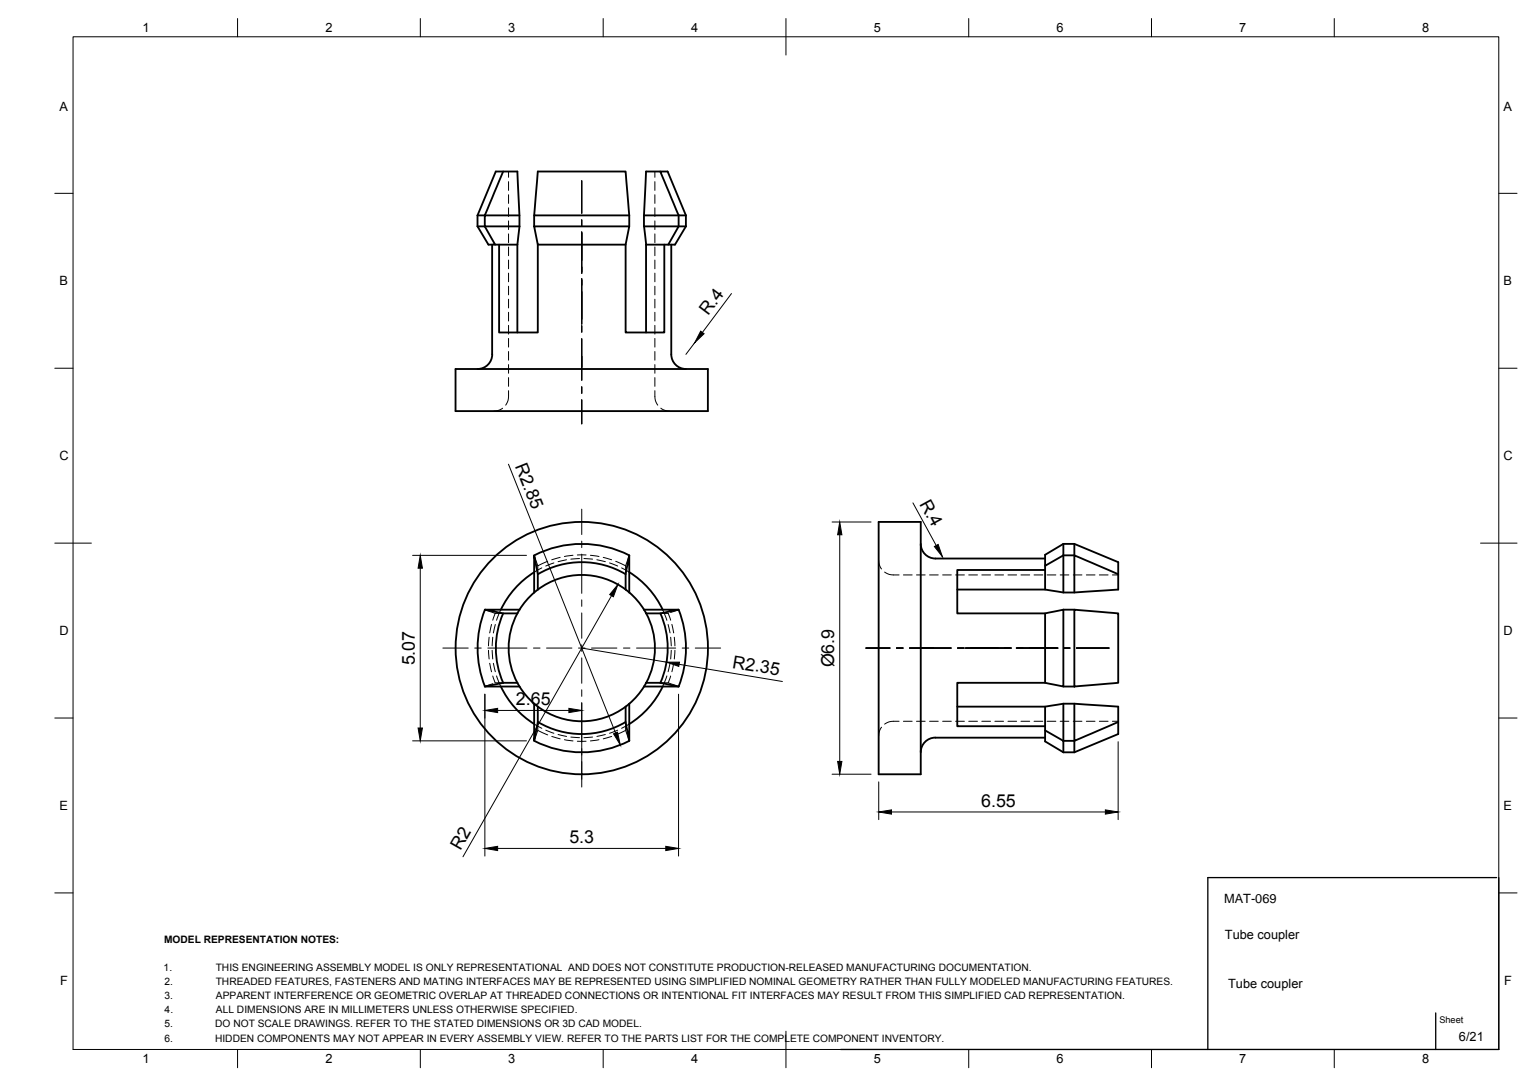
ISO-10303-21;
HEADER;
/* Generated by software containing ST-Developer
 * from STEP Tools, Inc. (www.steptools.com) 
 */

FILE_DESCRIPTION(
/* description */ ('CAx-IF Rec.Pracs.---Representation and Presentation of Product Manufa
cturing Information (PMI)---4.0---2014-10-13'),
/* implementation_level */ '2;1');

FILE_NAME(
/* name */ 'Tube coupler.step',
/* time_stamp */ '2026-10-24T15:08:39-07:00',
/* author */ (''),
/* organization */ (''),
/* preprocessor_version */ 'ST-DEVELOPER v20.2',
/* originating_system */ 'Autodesk Translation Framework v15.17.0.0',
/* authorisation */ '');

FILE_SCHEMA (('AP242_MANAGED_MODEL_BASED_3D_ENGINEERING_MIM_LF { 1 0 10303 442 2 1 4 }'));
ENDSEC;

DATA;
#10=MECHANICAL_DESIGN_GEOMETRIC_PRESENTATION_REPRESENTATION('',(#823),#50081);
#605=CONICAL_SURFACE('',#10189,0.0026,0.394791119699761);
#606=CONICAL_SURFACE('',#10204,0.0026,0.394791119699761);
#607=CONICAL_SURFACE('',#10207,0.0026,0.394791119699761);
#608=CONICAL_SURFACE('',#10215,0.0027,0.540419500270585);
#609=CONICAL_SURFACE('',#10219,0.0027,0.540419500270585);
#610=CONICAL_SURFACE('',#10227,0.0027,0.540419500270585);
#611=CONICAL_SURFACE('',#10235,0.0027,0.540419500270585);
#612=CONICAL_SURFACE('',#10257,0.0026,0.394791119699761);
#665=(
BOUNDED_CURVE()
B_SPLINE_CURVE(2,(#13666,#13667,#13668),.UNSPECIFIED.,.F.,.F.)
B_SPLINE_CURVE_WITH_KNOTS((3,3),(0.,0.130388293175992),.UNSPECIFIED.)
CURVE()
GEOMETRIC_REPRESENTATION_ITEM()
RATIONAL_B_SPLINE_CURVE((1.,1.00525170247464,1.))
REPRESENTATION_ITEM('')
);
#666=(
BOUNDED_CURVE()
B_SPLINE_CURVE(2,(#13674,#13675,#13676),.UNSPECIFIED.,.F.,.F.)
B_SPLINE_CURVE_WITH_KNOTS((3,3),(0.,0.130388293175992),.UNSPECIFIED.)
CURVE()
GEOMETRIC_REPRESENTATION_ITEM()
RATIONAL_B_SPLINE_CURVE((1.,1.00525170247464,1.))
REPRESENTATION_ITEM('')
);
#667=(
BOUNDED_CURVE()
B_SPLINE_CURVE(2,(#13686,#13687,#13688),.UNSPECIFIED.,.F.,.F.)
B_SPLINE_CURVE_WITH_KNOTS((3,3),(0.,0.1309950991442),.UNSPECIFIED.)
CURVE()
GEOMETRIC_REPRESENTATION_ITEM()
RATIONAL_B_SPLINE_CURVE((1.,1.00582981008257,1.))
REPRESENTATION_ITEM('')
);
#668=(
BOUNDED_CURVE()
B_SPLINE_CURVE(2,(#13697,#13698,#13699),.UNSPECIFIED.,.F.,.F.)
B_SPLINE_CURVE_WITH_KNOTS((3,3),(0.,0.1309950991442),.UNSPECIFIED.)
CURVE()
GEOMETRIC_REPRESENTATION_ITEM()
RATIONAL_B_SPLINE_CURVE((1.,1.00582981008257,1.))
REPRESENTATION_ITEM('')
);
#669=(
BOUNDED_CURVE()
B_SPLINE_CURVE(2,(#13708,#13709,#13710),.UNSPECIFIED.,.F.,.F.)
B_SPLINE_CURVE_WITH_KNOTS((3,3),(0.,0.1309950991442),.UNSPECIFIED.)
CURVE()
GEOMETRIC_REPRESENTATION_ITEM()
RATIONAL_B_SPLINE_CURVE((1.,1.00582981008257,1.))
REPRESENTATION_ITEM('')
);
#670=(
BOUNDED_CURVE()
B_SPLINE_CURVE(2,(#13715,#13716,#13717),.UNSPECIFIED.,.F.,.F.)
B_SPLINE_CURVE_WITH_KNOTS((3,3),(0.,0.130388293175992),.UNSPECIFIED.)
CURVE()
GEOMETRIC_REPRESENTATION_ITEM()
RATIONAL_B_SPLINE_CURVE((1.,1.00525170247464,1.))
REPRESENTATION_ITEM('')
);
#671=(
BOUNDED_CURVE()
B_SPLINE_CURVE(2,(#13727,#13728,#13729),.UNSPECIFIED.,.F.,.F.)
B_SPLINE_CURVE_WITH_KNOTS((3,3),(0.,0.130388293175992),.UNSPECIFIED.)
CURVE()
GEOMETRIC_REPRESENTATION_ITEM()
RATIONAL_B_SPLINE_CURVE((1.,1.00525170247464,1.))
REPRESENTATION_ITEM('')
);
#672=(
BOUNDED_CURVE()
B_SPLINE_CURVE(2,(#13732,#13733,#13734),.UNSPECIFIED.,.F.,.F.)
B_SPLINE_CURVE_WITH_KNOTS((3,3),(0.,0.1309950991442),.UNSPECIFIED.)
CURVE()
GEOMETRIC_REPRESENTATION_ITEM()
RATIONAL_B_SPLINE_CURVE((1.,1.00582981008257,1.))
REPRESENTATION_ITEM('')
);
#673=(
BOUNDED_CURVE()
B_SPLINE_CURVE(2,(#13762,#13763,#13764),.UNSPECIFIED.,.F.,.F.)
B_SPLINE_CURVE_WITH_KNOTS((3,3),(0.13740622471284,0.194564395432606),
 .UNSPECIFIED.)
CURVE()
GEOMETRIC_REPRESENTATION_ITEM()
RATIONAL_B_SPLINE_CURVE((1.0210752443686,1.02155284321629,1.018780946918))
REPRESENTATION_ITEM('')
);
#674=(
BOUNDED_CURVE()
B_SPLINE_CURVE(2,(#13772,#13773,#13774),.UNSPECIFIED.,.F.,.F.)
B_SPLINE_CURVE_WITH_KNOTS((3,3),(-0.194564395432341,-0.137406224712621),
 .UNSPECIFIED.)
CURVE()
GEOMETRIC_REPRESENTATION_ITEM()
RATIONAL_B_SPLINE_CURVE((1.01878094691633,1.02155284321435,1.02107524436669))
REPRESENTATION_ITEM('')
);
#675=(
BOUNDED_CURVE()
B_SPLINE_CURVE(2,(#13806,#13807,#13808),.UNSPECIFIED.,.F.,.F.)
B_SPLINE_CURVE_WITH_KNOTS((3,3),(0.137406224811474,0.19456439553049),
 .UNSPECIFIED.)
CURVE()
GEOMETRIC_REPRESENTATION_ITEM()
RATIONAL_B_SPLINE_CURVE((1.02107524478079,1.02155284363217,1.01878094727436))
REPRESENTATION_ITEM('')
);
#676=(
BOUNDED_CURVE()
B_SPLINE_CURVE(2,(#13815,#13816,#13817),.UNSPECIFIED.,.F.,.F.)
B_SPLINE_CURVE_WITH_KNOTS((3,3),(-0.194564395470828,-0.137406224751148),
 .UNSPECIFIED.)
CURVE()
GEOMETRIC_REPRESENTATION_ITEM()
RATIONAL_B_SPLINE_CURVE((1.01878094706027,1.02155284338227,1.02107524453305))
REPRESENTATION_ITEM('')
);
#687=ELLIPSE('',#10162,0.0240831891575954,0.00200000000001);
#688=ELLIPSE('',#10163,0.0101980390271974,0.00200000000001);
#689=ELLIPSE('',#10165,0.0101980390271974,0.00200000000001);
#690=ELLIPSE('',#10166,0.0240831891575954,0.00200000000001);
#691=ELLIPSE('',#10168,0.0240831891575954,0.00200000000001);
#692=ELLIPSE('',#10169,0.0101980390271974,0.00200000000001);
#693=ELLIPSE('',#10171,0.0101980390271974,0.00200000000001);
#694=ELLIPSE('',#10172,0.0240831891575954,0.00200000000001);
#695=ELLIPSE('',#10174,0.0240831891575954,0.00200000000001);
#696=ELLIPSE('',#10175,0.0101980390271974,0.00200000000001);
#697=ELLIPSE('',#10177,0.0101980390271974,0.00200000000001);
#698=ELLIPSE('',#10178,0.0240831891575954,0.00200000000001);
#699=ELLIPSE('',#10180,0.0240831891575954,0.00200000000001);
#700=ELLIPSE('',#10181,0.0101980390271974,0.00200000000001);
#701=ELLIPSE('',#10183,0.0101980390271974,0.00200000000001);
#702=ELLIPSE('',#10184,0.0240831891575954,0.00200000000001);
#710=FACE_BOUND('',#1658,.T.);
#711=FACE_BOUND('',#1663,.T.);
#771=TOROIDAL_SURFACE('',#10140,0.00285,0.0004);
#772=TOROIDAL_SURFACE('',#10156,0.0024,0.0004);
#783=SHAPE_REPRESENTATION_RELATIONSHIP('SRR','None',#50151,#803);
#803=ADVANCED_BREP_SHAPE_REPRESENTATION('',(#843),#50064);
#823=STYLED_ITEM('',(#50260),#843);
#843=MANIFOLD_SOLID_BREP('Body1',#9868);
#866=PLANE('',#10144);
#867=PLANE('',#10186);
#868=PLANE('',#10188);
#869=PLANE('',#10192);
#870=PLANE('',#10193);
#871=PLANE('',#10194);
#872=PLANE('',#10195);
#873=PLANE('',#10197);
#874=PLANE('',#10198);
#875=PLANE('',#10200);
#876=PLANE('',#10201);
#877=PLANE('',#10202);
#878=PLANE('',#10206);
#879=PLANE('',#10209);
#880=PLANE('',#10210);
#881=PLANE('',#10211);
#882=PLANE('',#10213);
#883=PLANE('',#10218);
#884=PLANE('',#10222);
#885=PLANE('',#10223);
#886=PLANE('',#10224);
#887=PLANE('',#10225);
#888=PLANE('',#10231);
#889=PLANE('',#10232);
#890=PLANE('',#10233);
#891=PLANE('',#10234);
#892=PLANE('',#10238);
#893=PLANE('',#10239);
#894=PLANE('',#10240);
#895=PLANE('',#10241);
#896=PLANE('',#10242);
#897=PLANE('',#10243);
#898=PLANE('',#10244);
#899=PLANE('',#10245);
#900=PLANE('',#10246);
#901=PLANE('',#10247);
#902=PLANE('',#10248);
#903=PLANE('',#10249);
#904=PLANE('',#10250);
#905=PLANE('',#10251);
#906=PLANE('',#10252);
#907=PLANE('',#10254);
#908=PLANE('',#10256);
#909=PLANE('',#10260);
#910=PLANE('',#10262);
#911=PLANE('',#10264);
#1115=FACE_OUTER_BOUND('',#1656,.T.);
#1116=FACE_OUTER_BOUND('',#1657,.T.);
#1117=FACE_OUTER_BOUND('',#1659,.T.);
#1118=FACE_OUTER_BOUND('',#1660,.T.);
#1119=FACE_OUTER_BOUND('',#1661,.T.);
#1120=FACE_OUTER_BOUND('',#1662,.T.);
#1121=FACE_OUTER_BOUND('',#1664,.T.);
#1122=FACE_OUTER_BOUND('',#1665,.T.);
#1123=FACE_OUTER_BOUND('',#1666,.T.);
#1124=FACE_OUTER_BOUND('',#1667,.T.);
#1125=FACE_OUTER_BOUND('',#1668,.T.);
#1126=FACE_OUTER_BOUND('',#1669,.T.);
#1127=FACE_OUTER_BOUND('',#1670,.T.);
#1128=FACE_OUTER_BOUND('',#1671,.T.);
#1129=FACE_OUTER_BOUND('',#1672,.T.);
#1130=FACE_OUTER_BOUND('',#1673,.T.);
#1131=FACE_OUTER_BOUND('',#1674,.T.);
#1132=FACE_OUTER_BOUND('',#1675,.T.);
#1133=FACE_OUTER_BOUND('',#1676,.T.);
#1134=FACE_OUTER_BOUND('',#1677,.T.);
#1135=FACE_OUTER_BOUND('',#1678,.T.);
#1136=FACE_OUTER_BOUND('',#1679,.T.);
#1137=FACE_OUTER_BOUND('',#1680,.T.);
#1138=FACE_OUTER_BOUND('',#1681,.T.);
#1139=FACE_OUTER_BOUND('',#1682,.T.);
#1140=FACE_OUTER_BOUND('',#1683,.T.);
#1141=FACE_OUTER_BOUND('',#1684,.T.);
#1142=FACE_OUTER_BOUND('',#1685,.T.);
#1143=FACE_OUTER_BOUND('',#1686,.T.);
#1144=FACE_OUTER_BOUND('',#1687,.T.);
#1145=FACE_OUTER_BOUND('',#1688,.T.);
#1146=FACE_OUTER_BOUND('',#1689,.T.);
#1147=FACE_OUTER_BOUND('',#1690,.T.);
#1148=FACE_OUTER_BOUND('',#1691,.T.);
#1149=FACE_OUTER_BOUND('',#1692,.T.);
#1150=FACE_OUTER_BOUND('',#1693,.T.);
#1151=FACE_OUTER_BOUND('',#1694,.T.);
#1152=FACE_OUTER_BOUND('',#1695,.T.);
#1153=FACE_OUTER_BOUND('',#1696,.T.);
#1154=FACE_OUTER_BOUND('',#1697,.T.);
#1155=FACE_OUTER_BOUND('',#1698,.T.);
#1156=FACE_OUTER_BOUND('',#1699,.T.);
#1157=FACE_OUTER_BOUND('',#1700,.T.);
#1158=FACE_OUTER_BOUND('',#1701,.T.);
#1159=FACE_OUTER_BOUND('',#1702,.T.);
#1160=FACE_OUTER_BOUND('',#1703,.T.);
#1161=FACE_OUTER_BOUND('',#1704,.T.);
#1162=FACE_OUTER_BOUND('',#1705,.T.);
#1163=FACE_OUTER_BOUND('',#1706,.T.);
#1164=FACE_OUTER_BOUND('',#1707,.T.);
#1165=FACE_OUTER_BOUND('',#1708,.T.);
#1166=FACE_OUTER_BOUND('',#1709,.T.);
#1167=FACE_OUTER_BOUND('',#1710,.T.);
#1168=FACE_OUTER_BOUND('',#1711,.T.);
#1169=FACE_OUTER_BOUND('',#1712,.T.);
#1170=FACE_OUTER_BOUND('',#1713,.T.);
#1171=FACE_OUTER_BOUND('',#1714,.T.);
#1172=FACE_OUTER_BOUND('',#1715,.T.);
#1173=FACE_OUTER_BOUND('',#1716,.T.);
#1174=FACE_OUTER_BOUND('',#1717,.T.);
#1175=FACE_OUTER_BOUND('',#1718,.T.);
#1176=FACE_OUTER_BOUND('',#1719,.T.);
#1177=FACE_OUTER_BOUND('',#1720,.T.);
#1656=EDGE_LOOP('',(#6268,#6269,#6270,#6271));
#1657=EDGE_LOOP('',(#6272));
#1658=EDGE_LOOP('',(#6273));
#1659=EDGE_LOOP('',(#6274,#6275,#6276,#6277,#6278,#6279,#6280,#6281,#6282,
#6283,#6284,#6285,#6286,#6287,#6288,#6289,#6290,#6291,#6292,#6293));
#1660=EDGE_LOOP('',(#6294,#6295,#6296,#6297));
#1661=EDGE_LOOP('',(#6298,#6299,#6300,#6301,#6302,#6303,#6304,#6305,#6306,
#6307,#6308,#6309,#6310,#6311,#6312,#6313,#6314,#6315,#6316,#6317,#6318,
#6319,#6320,#6321,#6322,#6323,#6324,#6325,#6326,#6327,#6328,#6329,#6330,
#6331,#6332,#6333,#6334,#6335,#6336,#6337,#6338,#6339,#6340,#6341));
#1662=EDGE_LOOP('',(#6342));
#1663=EDGE_LOOP('',(#6343));
#1664=EDGE_LOOP('',(#6344,#6345,#6346,#6347));
#1665=EDGE_LOOP('',(#6348,#6349,#6350,#6351));
#1666=EDGE_LOOP('',(#6352,#6353,#6354,#6355));
#1667=EDGE_LOOP('',(#6356,#6357,#6358,#6359));
#1668=EDGE_LOOP('',(#6360,#6361,#6362,#6363));
#1669=EDGE_LOOP('',(#6364,#6365,#6366,#6367));
#1670=EDGE_LOOP('',(#6368,#6369,#6370,#6371));
#1671=EDGE_LOOP('',(#6372,#6373,#6374,#6375,#6376));
#1672=EDGE_LOOP('',(#6377,#6378,#6379,#6380));
#1673=EDGE_LOOP('',(#6381,#6382,#6383,#6384));
#1674=EDGE_LOOP('',(#6385,#6386,#6387,#6388));
#1675=EDGE_LOOP('',(#6389,#6390,#6391,#6392));
#1676=EDGE_LOOP('',(#6393,#6394,#6395,#6396));
#1677=EDGE_LOOP('',(#6397,#6398,#6399,#6400));
#1678=EDGE_LOOP('',(#6401,#6402,#6403,#6404));
#1679=EDGE_LOOP('',(#6405,#6406,#6407,#6408));
#1680=EDGE_LOOP('',(#6409,#6410,#6411,#6412,#6413));
#1681=EDGE_LOOP('',(#6414,#6415,#6416,#6417));
#1682=EDGE_LOOP('',(#6418,#6419,#6420,#6421));
#1683=EDGE_LOOP('',(#6422,#6423,#6424,#6425,#6426));
#1684=EDGE_LOOP('',(#6427,#6428,#6429,#6430));
#1685=EDGE_LOOP('',(#6431,#6432,#6433,#6434));
#1686=EDGE_LOOP('',(#6435,#6436,#6437,#6438,#6439));
#1687=EDGE_LOOP('',(#6440,#6441,#6442,#6443));
#1688=EDGE_LOOP('',(#6444,#6445,#6446,#6447,#6448));
#1689=EDGE_LOOP('',(#6449,#6450,#6451,#6452));
#1690=EDGE_LOOP('',(#6453,#6454,#6455,#6456,#6457));
#1691=EDGE_LOOP('',(#6458,#6459,#6460,#6461,#6462));
#1692=EDGE_LOOP('',(#6463,#6464,#6465,#6466));
#1693=EDGE_LOOP('',(#6467,#6468,#6469,#6470,#6471));
#1694=EDGE_LOOP('',(#6472,#6473,#6474,#6475));
#1695=EDGE_LOOP('',(#6476,#6477,#6478,#6479));
#1696=EDGE_LOOP('',(#6480,#6481,#6482,#6483,#6484));
#1697=EDGE_LOOP('',(#6485,#6486,#6487,#6488,#6489));
#1698=EDGE_LOOP('',(#6490,#6491,#6492,#6493));
#1699=EDGE_LOOP('',(#6494,#6495,#6496,#6497));
#1700=EDGE_LOOP('',(#6498,#6499,#6500,#6501));
#1701=EDGE_LOOP('',(#6502,#6503,#6504,#6505));
#1702=EDGE_LOOP('',(#6506,#6507,#6508,#6509));
#1703=EDGE_LOOP('',(#6510,#6511,#6512,#6513));
#1704=EDGE_LOOP('',(#6514,#6515,#6516,#6517));
#1705=EDGE_LOOP('',(#6518,#6519,#6520,#6521));
#1706=EDGE_LOOP('',(#6522,#6523,#6524,#6525));
#1707=EDGE_LOOP('',(#6526,#6527,#6528,#6529));
#1708=EDGE_LOOP('',(#6530,#6531,#6532,#6533));
#1709=EDGE_LOOP('',(#6534,#6535,#6536,#6537));
#1710=EDGE_LOOP('',(#6538,#6539,#6540,#6541));
#1711=EDGE_LOOP('',(#6542,#6543,#6544,#6545));
#1712=EDGE_LOOP('',(#6546,#6547,#6548,#6549));
#1713=EDGE_LOOP('',(#6550,#6551,#6552,#6553));
#1714=EDGE_LOOP('',(#6554,#6555,#6556,#6557));
#1715=EDGE_LOOP('',(#6558,#6559,#6560,#6561));
#1716=EDGE_LOOP('',(#6562,#6563,#6564,#6565));
#1717=EDGE_LOOP('',(#6566,#6567,#6568,#6569));
#1718=EDGE_LOOP('',(#6570,#6571,#6572,#6573));
#1719=EDGE_LOOP('',(#6574,#6575,#6576,#6577));
#1720=EDGE_LOOP('',(#6578,#6579,#6580,#6581));
#2248=LINE('',#13538,#2826);
#2249=LINE('',#13542,#2827);
#2250=LINE('',#13546,#2828);
#2251=LINE('',#13550,#2829);
#2252=LINE('',#13554,#2830);
#2253=LINE('',#13558,#2831);
#2254=LINE('',#13562,#2832);
#2255=LINE('',#13566,#2833);
#2256=LINE('',#13568,#2834);
#2257=LINE('',#13577,#2835);
#2258=LINE('',#13583,#2836);
#2259=LINE('',#13587,#2837);
#2260=LINE('',#13591,#2838);
#2261=LINE('',#13595,#2839);
#2262=LINE('',#13603,#2840);
#2263=LINE('',#13607,#2841);
#2264=LINE('',#13611,#2842);
#2265=LINE('',#13615,#2843);
#2266=LINE('',#13623,#2844);
#2267=LINE('',#13627,#2845);
#2268=LINE('',#13631,#2846);
#2269=LINE('',#13635,#2847);
#2270=LINE('',#13643,#2848);
#2271=LINE('',#13647,#2849);
#2272=LINE('',#13651,#2850);
#2273=LINE('',#13655,#2851);
#2274=LINE('',#13664,#2852);
#2275=LINE('',#13669,#2853);
#2276=LINE('',#13679,#2854);
#2277=LINE('',#13681,#2855);
#2278=LINE('',#13684,#2856);
#2279=LINE('',#13689,#2857);
#2280=LINE('',#13692,#2858);
#2281=LINE('',#13700,#2859);
#2282=LINE('',#13701,#2860);
#2283=LINE('',#13705,#2861);
#2284=LINE('',#13711,#2862);
#2285=LINE('',#13718,#2863);
#2286=LINE('',#13719,#2864);
#2287=LINE('',#13723,#2865);
#2288=LINE('',#13735,#2866);
#2289=LINE('',#13739,#2867);
#2290=LINE('',#13742,#2868);
#2291=LINE('',#13743,#2869);
#2292=LINE('',#13746,#2870);
#2293=LINE('',#13749,#2871);
#2294=LINE('',#13750,#2872);
#2295=LINE('',#13754,#2873);
#2296=LINE('',#13765,#2874);
#2297=LINE('',#13766,#2875);
#2298=LINE('',#13767,#2876);
#2299=LINE('',#13777,#2877);
#2300=LINE('',#13779,#2878);
#2301=LINE('',#13780,#2879);
#2302=LINE('',#13782,#2880);
#2303=LINE('',#13787,#2881);
#2304=LINE('',#13788,#2882);
#2305=LINE('',#13789,#2883);
#2306=LINE('',#13797,#2884);
#2307=LINE('',#13799,#2885);
#2308=LINE('',#13800,#2886);
#2309=LINE('',#13802,#2887);
#2310=LINE('',#13809,#2888);
#2311=LINE('',#13810,#2889);
#2312=LINE('',#13811,#2890);
#2313=LINE('',#13820,#2891);
#2314=LINE('',#13822,#2892);
#2315=LINE('',#13823,#2893);
#2316=LINE('',#13825,#2894);
#2317=LINE('',#13827,#2895);
#2318=LINE('',#13829,#2896);
#2319=LINE('',#13831,#2897);
#2320=LINE('',#13833,#2898);
#2321=LINE('',#13835,#2899);
#2322=LINE('',#13837,#2900);
#2323=LINE('',#13839,#2901);
#2324=LINE('',#13841,#2902);
#2325=LINE('',#13847,#2903);
#2326=LINE('',#13849,#2904);
#2327=LINE('',#13851,#2905);
#2328=LINE('',#13856,#2906);
#2329=LINE('',#13859,#2907);
#2330=LINE('',#13862,#2908);
#2826=VECTOR('',#11124,1.);
#2827=VECTOR('',#11127,1.);
#2828=VECTOR('',#11130,1.);
#2829=VECTOR('',#11133,1.);
#2830=VECTOR('',#11136,1.);
#2831=VECTOR('',#11139,1.);
#2832=VECTOR('',#11142,1.);
#2833=VECTOR('',#11145,1.);
#2834=VECTOR('',#11148,0.00245);
#2835=VECTOR('',#11159,0.002);
#2836=VECTOR('',#11164,1.);
#2837=VECTOR('',#11167,1.);
#2838=VECTOR('',#11170,1.);
#2839=VECTOR('',#11173,1.);
#2840=VECTOR('',#11180,1.);
#2841=VECTOR('',#11183,1.);
#2842=VECTOR('',#11186,1.);
#2843=VECTOR('',#11189,1.);
#2844=VECTOR('',#11196,1.);
#2845=VECTOR('',#11199,1.);
#2846=VECTOR('',#11202,1.);
#2847=VECTOR('',#11205,1.);
#2848=VECTOR('',#11212,1.);
#2849=VECTOR('',#11215,1.);
#2850=VECTOR('',#11218,1.);
#2851=VECTOR('',#11221,1.);
#2852=VECTOR('',#11232,1.);
#2853=VECTOR('',#11233,1.);
#2854=VECTOR('',#11242,1.);
#2855=VECTOR('',#11245,1.);
#2856=VECTOR('',#11248,1.);
#2857=VECTOR('',#11249,1.);
#2858=VECTOR('',#11252,1.);
#2859=VECTOR('',#11257,1.);
#2860=VECTOR('',#11258,1.);
#2861=VECTOR('',#11263,1.);
#2862=VECTOR('',#11266,1.);
#2863=VECTOR('',#11269,1.);
#2864=VECTOR('',#11270,1.);
#2865=VECTOR('',#11275,1.);
#2866=VECTOR('',#11282,1.);
#2867=VECTOR('',#11289,1.);
#2868=VECTOR('',#11292,1.);
#2869=VECTOR('',#11293,1.);
#2870=VECTOR('',#11296,1.);
#2871=VECTOR('',#11299,1.);
#2872=VECTOR('',#11300,1.);
#2873=VECTOR('',#11305,1.);
#2874=VECTOR('',#11314,1.);
#2875=VECTOR('',#11315,1.);
#2876=VECTOR('',#11316,1.);
#2877=VECTOR('',#11325,1.);
#2878=VECTOR('',#11328,1.);
#2879=VECTOR('',#11329,1.);
#2880=VECTOR('',#11332,1.);
#2881=VECTOR('',#11337,1.);
#2882=VECTOR('',#11338,1.);
#2883=VECTOR('',#11339,1.);
#2884=VECTOR('',#11350,1.);
#2885=VECTOR('',#11353,1.);
#2886=VECTOR('',#11354,1.);
#2887=VECTOR('',#11357,1.);
#2888=VECTOR('',#11360,1.);
#2889=VECTOR('',#11361,1.);
#2890=VECTOR('',#11362,1.);
#2891=VECTOR('',#11371,1.);
#2892=VECTOR('',#11374,1.);
#2893=VECTOR('',#11375,1.);
#2894=VECTOR('',#11378,1.);
#2895=VECTOR('',#11381,1.);
#2896=VECTOR('',#11384,1.);
#2897=VECTOR('',#11387,1.);
#2898=VECTOR('',#11390,1.);
#2899=VECTOR('',#11393,1.);
#2900=VECTOR('',#11396,1.);
#2901=VECTOR('',#11399,1.);
#2902=VECTOR('',#11402,1.);
#2903=VECTOR('',#11413,0.00345);
#2904=VECTOR('',#11416,1.);
#2905=VECTOR('',#11419,1.);
#2906=VECTOR('',#11428,1.);
#2907=VECTOR('',#11433,1.);
#2908=VECTOR('',#11438,1.);
#3415=CIRCLE('',#10141,0.0028500000000131);
#3416=CIRCLE('',#10142,0.0004);
#3417=CIRCLE('',#10143,0.00245000000001309);
#3418=CIRCLE('',#10145,0.00345000000001);
#3419=CIRCLE('',#10147,0.00245000000001);
#3420=CIRCLE('',#10148,0.00245000000001);
#3421=CIRCLE('',#10149,0.00245000000001);
#3422=CIRCLE('',#10150,0.00245000000001);
#3423=CIRCLE('',#10151,0.00245000000001);
#3424=CIRCLE('',#10152,0.00245000000001);
#3425=CIRCLE('',#10153,0.00245000000001);
#3426=CIRCLE('',#10154,0.00245000000001);
#3427=CIRCLE('',#10155,0.00245000000001);
#3428=CIRCLE('',#10157,0.00200000000001);
#3429=CIRCLE('',#10158,0.0004);
#3430=CIRCLE('',#10159,0.00240000000001);
#3431=CIRCLE('',#10161,0.00200000000001);
#3432=CIRCLE('',#10164,0.00200000000001);
#3433=CIRCLE('',#10167,0.00200000000001);
#3434=CIRCLE('',#10170,0.00200000000001);
#3435=CIRCLE('',#10173,0.00200000000001);
#3436=CIRCLE('',#10176,0.00200000000001);
#3437=CIRCLE('',#10179,0.00200000000001);
#3438=CIRCLE('',#10182,0.00200000000001);
#3439=CIRCLE('',#10185,0.00200000000001);
#3440=CIRCLE('',#10187,0.00345000000001);
#3441=CIRCLE('',#10190,0.00235000000001);
#3442=CIRCLE('',#10191,0.00285000000001);
#3443=CIRCLE('',#10196,0.00235000000001);
#3444=CIRCLE('',#10199,0.00235000000001);
#3445=CIRCLE('',#10203,0.00235000000001);
#3446=CIRCLE('',#10205,0.00285000000001);
#3447=CIRCLE('',#10208,0.00285000000001);
#3448=CIRCLE('',#10212,0.481704687282423);
#3449=CIRCLE('',#10214,0.00255000000001);
#3450=CIRCLE('',#10216,0.00285000000001);
#3451=CIRCLE('',#10217,0.481704687282423);
#3452=CIRCLE('',#10220,0.00255000000001);
#3453=CIRCLE('',#10221,0.00285000000001);
#3454=CIRCLE('',#10226,0.481704687282423);
#3455=CIRCLE('',#10228,0.00255000000001);
#3456=CIRCLE('',#10229,0.481704687282423);
#3457=CIRCLE('',#10230,0.00285000000001);
#3458=CIRCLE('',#10236,0.00255000000001);
#3459=CIRCLE('',#10237,0.00285000000001);
#3460=CIRCLE('',#10258,0.00285000000001);
#3786=VERTEX_POINT('',#13525);
#3787=VERTEX_POINT('',#13527);
#3788=VERTEX_POINT('',#13531);
#3789=VERTEX_POINT('',#13534);
#3790=VERTEX_POINT('',#13535);
#3791=VERTEX_POINT('',#13537);
#3792=VERTEX_POINT('',#13539);
#3793=VERTEX_POINT('',#13541);
#3794=VERTEX_POINT('',#13543);
#3795=VERTEX_POINT('',#13545);
#3796=VERTEX_POINT('',#13547);
#3797=VERTEX_POINT('',#13549);
#3798=VERTEX_POINT('',#13551);
#3799=VERTEX_POINT('',#13553);
#3800=VERTEX_POINT('',#13555);
#3801=VERTEX_POINT('',#13557);
#3802=VERTEX_POINT('',#13559);
#3803=VERTEX_POINT('',#13561);
#3804=VERTEX_POINT('',#13563);
#3805=VERTEX_POINT('',#13565);
#3806=VERTEX_POINT('',#13570);
#3807=VERTEX_POINT('',#13572);
#3808=VERTEX_POINT('',#13576);
#3809=VERTEX_POINT('',#13578);
#3810=VERTEX_POINT('',#13580);
#3811=VERTEX_POINT('',#13582);
#3812=VERTEX_POINT('',#13584);
#3813=VERTEX_POINT('',#13586);
#3814=VERTEX_POINT('',#13588);
#3815=VERTEX_POINT('',#13590);
#3816=VERTEX_POINT('',#13592);
#3817=VERTEX_POINT('',#13594);
#3818=VERTEX_POINT('',#13596);
#3819=VERTEX_POINT('',#13598);
#3820=VERTEX_POINT('',#13600);
#3821=VERTEX_POINT('',#13602);
#3822=VERTEX_POINT('',#13604);
#3823=VERTEX_POINT('',#13606);
#3824=VERTEX_POINT('',#13608);
#3825=VERTEX_POINT('',#13610);
#3826=VERTEX_POINT('',#13612);
#3827=VERTEX_POINT('',#13614);
#3828=VERTEX_POINT('',#13616);
#3829=VERTEX_POINT('',#13618);
#3830=VERTEX_POINT('',#13620);
#3831=VERTEX_POINT('',#13622);
#3832=VERTEX_POINT('',#13624);
#3833=VERTEX_POINT('',#13626);
#3834=VERTEX_POINT('',#13628);
#3835=VERTEX_POINT('',#13630);
#3836=VERTEX_POINT('',#13632);
#3837=VERTEX_POINT('',#13634);
#3838=VERTEX_POINT('',#13636);
#3839=VERTEX_POINT('',#13638);
#3840=VERTEX_POINT('',#13640);
#3841=VERTEX_POINT('',#13642);
#3842=VERTEX_POINT('',#13644);
#3843=VERTEX_POINT('',#13646);
#3844=VERTEX_POINT('',#13648);
#3845=VERTEX_POINT('',#13650);
#3846=VERTEX_POINT('',#13652);
#3847=VERTEX_POINT('',#13654);
#3848=VERTEX_POINT('',#13656);
#3849=VERTEX_POINT('',#13660);
#3850=VERTEX_POINT('',#13663);
#3851=VERTEX_POINT('',#13665);
#3852=VERTEX_POINT('',#13671);
#3853=VERTEX_POINT('',#13673);
#3854=VERTEX_POINT('',#13683);
#3855=VERTEX_POINT('',#13685);
#3856=VERTEX_POINT('',#13691);
#3857=VERTEX_POINT('',#13695);
#3858=VERTEX_POINT('',#13696);
#3859=VERTEX_POINT('',#13703);
#3860=VERTEX_POINT('',#13707);
#3861=VERTEX_POINT('',#13713);
#3862=VERTEX_POINT('',#13714);
#3863=VERTEX_POINT('',#13721);
#3864=VERTEX_POINT('',#13725);
#3865=VERTEX_POINT('',#13731);
#3866=VERTEX_POINT('',#13741);
#3867=VERTEX_POINT('',#13745);
#3868=VERTEX_POINT('',#13747);
#3869=VERTEX_POINT('',#13752);
#3870=VERTEX_POINT('',#13756);
#3871=VERTEX_POINT('',#13760);
#3872=VERTEX_POINT('',#13761);
#3873=VERTEX_POINT('',#13769);
#3874=VERTEX_POINT('',#13771);
#3875=VERTEX_POINT('',#13784);
#3876=VERTEX_POINT('',#13785);
#3877=VERTEX_POINT('',#13791);
#3878=VERTEX_POINT('',#13793);
#3879=VERTEX_POINT('',#13804);
#3880=VERTEX_POINT('',#13805);
#3881=VERTEX_POINT('',#13813);
#4787=EDGE_CURVE('',#3786,#3786,#3415,.T.);
#4788=EDGE_CURVE('',#3786,#3787,#3416,.T.);
#4789=EDGE_CURVE('',#3787,#3787,#3417,.T.);
#4790=EDGE_CURVE('',#3788,#3788,#3418,.T.);
#4791=EDGE_CURVE('',#3789,#3790,#3419,.T.);
#4792=EDGE_CURVE('',#3791,#3789,#2248,.T.);
#4793=EDGE_CURVE('',#3792,#3791,#3420,.T.);
#4794=EDGE_CURVE('',#3792,#3793,#2249,.T.);
#4795=EDGE_CURVE('',#3794,#3793,#3421,.T.);
#4796=EDGE_CURVE('',#3795,#3794,#2250,.T.);
#4797=EDGE_CURVE('',#3796,#3795,#3422,.T.);
#4798=EDGE_CURVE('',#3796,#3797,#2251,.T.);
#4799=EDGE_CURVE('',#3798,#3797,#3423,.T.);
#4800=EDGE_CURVE('',#3799,#3798,#2252,.T.);
#4801=EDGE_CURVE('',#3800,#3799,#3424,.T.);
#4802=EDGE_CURVE('',#3800,#3801,#2253,.T.);
#4803=EDGE_CURVE('',#3802,#3801,#3425,.T.);
#4804=EDGE_CURVE('',#3803,#3802,#2254,.T.);
#4805=EDGE_CURVE('',#3804,#3803,#3426,.T.);
#4806=EDGE_CURVE('',#3804,#3805,#2255,.T.);
#4807=EDGE_CURVE('',#3790,#3805,#3427,.T.);
#4808=EDGE_CURVE('',#3790,#3787,#2256,.T.);
#4809=EDGE_CURVE('',#3806,#3806,#3428,.T.);
#4810=EDGE_CURVE('',#3806,#3807,#3429,.T.);
#4811=EDGE_CURVE('',#3807,#3807,#3430,.T.);
#4812=EDGE_CURVE('',#3806,#3808,#2257,.T.);
#4813=EDGE_CURVE('',#3809,#3808,#3431,.T.);
#4814=EDGE_CURVE('',#3810,#3809,#687,.T.);
#4815=EDGE_CURVE('',#3811,#3810,#2258,.T.);
#4816=EDGE_CURVE('',#3812,#3811,#688,.T.);
#4817=EDGE_CURVE('',#3813,#3812,#2259,.T.);
#4818=EDGE_CURVE('',#3814,#3813,#3432,.T.);
#4819=EDGE_CURVE('',#3814,#3815,#2260,.T.);
#4820=EDGE_CURVE('',#3816,#3815,#689,.T.);
#4821=EDGE_CURVE('',#3816,#3817,#2261,.T.);
#4822=EDGE_CURVE('',#3818,#3817,#690,.T.);
#4823=EDGE_CURVE('',#3819,#3818,#3433,.T.);
#4824=EDGE_CURVE('',#3820,#3819,#691,.T.);
#4825=EDGE_CURVE('',#3821,#3820,#2262,.T.);
#4826=EDGE_CURVE('',#3822,#3821,#692,.T.);
#4827=EDGE_CURVE('',#3823,#3822,#2263,.T.);
#4828=EDGE_CURVE('',#3824,#3823,#3434,.T.);
#4829=EDGE_CURVE('',#3824,#3825,#2264,.T.);
#4830=EDGE_CURVE('',#3826,#3825,#693,.T.);
#4831=EDGE_CURVE('',#3826,#3827,#2265,.T.);
#4832=EDGE_CURVE('',#3828,#3827,#694,.T.);
#4833=EDGE_CURVE('',#3829,#3828,#3435,.T.);
#4834=EDGE_CURVE('',#3830,#3829,#695,.T.);
#4835=EDGE_CURVE('',#3831,#3830,#2266,.T.);
#4836=EDGE_CURVE('',#3832,#3831,#696,.T.);
#4837=EDGE_CURVE('',#3833,#3832,#2267,.T.);
#4838=EDGE_CURVE('',#3834,#3833,#3436,.T.);
#4839=EDGE_CURVE('',#3834,#3835,#2268,.T.);
#4840=EDGE_CURVE('',#3836,#3835,#697,.T.);
#4841=EDGE_CURVE('',#3836,#3837,#2269,.T.);
#4842=EDGE_CURVE('',#3838,#3837,#698,.T.);
#4843=EDGE_CURVE('',#3839,#3838,#3437,.T.);
#4844=EDGE_CURVE('',#3840,#3839,#699,.T.);
#4845=EDGE_CURVE('',#3841,#3840,#2270,.T.);
#4846=EDGE_CURVE('',#3842,#3841,#700,.T.);
#4847=EDGE_CURVE('',#3843,#3842,#2271,.T.);
#4848=EDGE_CURVE('',#3844,#3843,#3438,.T.);
#4849=EDGE_CURVE('',#3844,#3845,#2272,.T.);
#4850=EDGE_CURVE('',#3846,#3845,#701,.T.);
#4851=EDGE_CURVE('',#3846,#3847,#2273,.T.);
#4852=EDGE_CURVE('',#3848,#3847,#702,.T.);
#4853=EDGE_CURVE('',#3808,#3848,#3439,.T.);
#4854=EDGE_CURVE('',#3849,#3849,#3440,.T.);
#4855=EDGE_CURVE('',#3839,#3850,#2274,.T.);
#4856=EDGE_CURVE('',#3850,#3851,#665,.T.);
#4857=EDGE_CURVE('',#3851,#3840,#2275,.T.);
#4858=EDGE_CURVE('',#3850,#3852,#3441,.T.);
#4859=EDGE_CURVE('',#3853,#3852,#666,.T.);
#4860=EDGE_CURVE('',#3853,#3851,#3442,.T.);
#4861=EDGE_CURVE('',#3852,#3838,#2276,.T.);
#4862=EDGE_CURVE('',#3837,#3853,#2277,.T.);
#4863=EDGE_CURVE('',#3829,#3854,#2278,.T.);
#4864=EDGE_CURVE('',#3854,#3855,#667,.T.);
#4865=EDGE_CURVE('',#3855,#3830,#2279,.T.);
#4866=EDGE_CURVE('',#3856,#3828,#2280,.T.);
#4867=EDGE_CURVE('',#3854,#3856,#3443,.T.);
#4868=EDGE_CURVE('',#3857,#3858,#668,.T.);
#4869=EDGE_CURVE('',#3858,#3848,#2281,.T.);
#4870=EDGE_CURVE('',#3847,#3857,#2282,.T.);
#4871=EDGE_CURVE('',#3859,#3858,#3444,.T.);
#4872=EDGE_CURVE('',#3809,#3859,#2283,.T.);
#4873=EDGE_CURVE('',#3859,#3860,#669,.T.);
#4874=EDGE_CURVE('',#3860,#3810,#2284,.T.);
#4875=EDGE_CURVE('',#3861,#3862,#670,.T.);
#4876=EDGE_CURVE('',#3862,#3818,#2285,.T.);
#4877=EDGE_CURVE('',#3817,#3861,#2286,.T.);
#4878=EDGE_CURVE('',#3863,#3862,#3445,.T.);
#4879=EDGE_CURVE('',#3819,#3863,#2287,.T.);
#4880=EDGE_CURVE('',#3861,#3864,#3446,.T.);
#4881=EDGE_CURVE('',#3863,#3864,#671,.T.);
#4882=EDGE_CURVE('',#3865,#3856,#672,.T.);
#4883=EDGE_CURVE('',#3827,#3865,#2288,.T.);
#4884=EDGE_CURVE('',#3865,#3855,#3447,.T.);
#4885=EDGE_CURVE('',#3864,#3820,#2289,.T.);
#4886=EDGE_CURVE('',#3866,#3864,#2290,.T.);
#4887=EDGE_CURVE('',#3821,#3866,#2291,.T.);
#4888=EDGE_CURVE('',#3831,#3867,#2292,.T.);
#4889=EDGE_CURVE('',#3867,#3868,#3448,.T.);
#4890=EDGE_CURVE('',#3868,#3797,#2293,.T.);
#4891=EDGE_CURVE('',#3797,#3832,#2294,.T.);
#4892=EDGE_CURVE('',#3869,#3868,#3449,.T.);
#4893=EDGE_CURVE('',#3798,#3869,#2295,.T.);
#4894=EDGE_CURVE('',#3867,#3870,#3450,.T.);
#4895=EDGE_CURVE('',#3869,#3870,#3451,.T.);
#4896=EDGE_CURVE('',#3871,#3872,#673,.T.);
#4897=EDGE_CURVE('',#3872,#3836,#2296,.T.);
#4898=EDGE_CURVE('',#3835,#3794,#2297,.T.);
#4899=EDGE_CURVE('',#3794,#3871,#2298,.T.);
#4900=EDGE_CURVE('',#3871,#3873,#3452,.T.);
#4901=EDGE_CURVE('',#3874,#3873,#674,.T.);
#4902=EDGE_CURVE('',#3874,#3872,#3453,.T.);
#4903=EDGE_CURVE('',#3873,#3793,#2299,.T.);
#4904=EDGE_CURVE('',#3841,#3874,#2300,.T.);
#4905=EDGE_CURVE('',#3793,#3842,#2301,.T.);
#4906=EDGE_CURVE('',#3874,#3851,#2302,.T.);
#4907=EDGE_CURVE('',#3875,#3876,#3454,.T.);
#4908=EDGE_CURVE('',#3876,#3846,#2303,.T.);
#4909=EDGE_CURVE('',#3845,#3789,#2304,.T.);
#4910=EDGE_CURVE('',#3789,#3875,#2305,.T.);
#4911=EDGE_CURVE('',#3875,#3877,#3455,.T.);
#4912=EDGE_CURVE('',#3878,#3877,#3456,.T.);
#4913=EDGE_CURVE('',#3878,#3876,#3457,.T.);
#4914=EDGE_CURVE('',#3877,#3805,#2306,.T.);
#4915=EDGE_CURVE('',#3811,#3878,#2307,.T.);
#4916=EDGE_CURVE('',#3805,#3812,#2308,.T.);
#4917=EDGE_CURVE('',#3878,#3860,#2309,.T.);
#4918=EDGE_CURVE('',#3879,#3880,#675,.T.);
#4919=EDGE_CURVE('',#3880,#3816,#2310,.T.);
#4920=EDGE_CURVE('',#3815,#3802,#2311,.T.);
#4921=EDGE_CURVE('',#3802,#3879,#2312,.T.);
#4922=EDGE_CURVE('',#3879,#3881,#3458,.T.);
#4923=EDGE_CURVE('',#3866,#3881,#676,.T.);
#4924=EDGE_CURVE('',#3866,#3880,#3459,.T.);
#4925=EDGE_CURVE('',#3881,#3801,#2313,.T.);
#4926=EDGE_CURVE('',#3870,#3826,#2314,.T.);
#4927=EDGE_CURVE('',#3825,#3798,#2315,.T.);
#4928=EDGE_CURVE('',#3801,#3822,#2316,.T.);
#4929=EDGE_CURVE('',#3795,#3834,#2317,.T.);
#4930=EDGE_CURVE('',#3843,#3792,#2318,.T.);
#4931=EDGE_CURVE('',#3799,#3824,#2319,.T.);
#4932=EDGE_CURVE('',#3833,#3796,#2320,.T.);
#4933=EDGE_CURVE('',#3791,#3844,#2321,.T.);
#4934=EDGE_CURVE('',#3813,#3804,#2322,.T.);
#4935=EDGE_CURVE('',#3803,#3814,#2323,.T.);
#4936=EDGE_CURVE('',#3823,#3800,#2324,.T.);
#4937=EDGE_CURVE('',#3788,#3849,#2325,.T.);
#4938=EDGE_CURVE('',#3867,#3855,#2326,.T.);
#4939=EDGE_CURVE('',#3870,#3865,#2327,.T.);
#4940=EDGE_CURVE('',#3857,#3860,#3460,.T.);
#4941=EDGE_CURVE('',#3876,#3857,#2328,.T.);
#4942=EDGE_CURVE('',#3880,#3861,#2329,.T.);
#4943=EDGE_CURVE('',#3872,#3853,#2330,.T.);
#6268=ORIENTED_EDGE('',*,*,#4787,.T.);
#6269=ORIENTED_EDGE('',*,*,#4788,.T.);
#6270=ORIENTED_EDGE('',*,*,#4789,.T.);
#6271=ORIENTED_EDGE('',*,*,#4788,.F.);
#6272=ORIENTED_EDGE('',*,*,#4790,.T.);
#6273=ORIENTED_EDGE('',*,*,#4787,.F.);
#6274=ORIENTED_EDGE('',*,*,#4791,.F.);
#6275=ORIENTED_EDGE('',*,*,#4792,.F.);
#6276=ORIENTED_EDGE('',*,*,#4793,.F.);
#6277=ORIENTED_EDGE('',*,*,#4794,.T.);
#6278=ORIENTED_EDGE('',*,*,#4795,.F.);
#6279=ORIENTED_EDGE('',*,*,#4796,.F.);
#6280=ORIENTED_EDGE('',*,*,#4797,.F.);
#6281=ORIENTED_EDGE('',*,*,#4798,.T.);
#6282=ORIENTED_EDGE('',*,*,#4799,.F.);
#6283=ORIENTED_EDGE('',*,*,#4800,.F.);
#6284=ORIENTED_EDGE('',*,*,#4801,.F.);
#6285=ORIENTED_EDGE('',*,*,#4802,.T.);
#6286=ORIENTED_EDGE('',*,*,#4803,.F.);
#6287=ORIENTED_EDGE('',*,*,#4804,.F.);
#6288=ORIENTED_EDGE('',*,*,#4805,.F.);
#6289=ORIENTED_EDGE('',*,*,#4806,.T.);
#6290=ORIENTED_EDGE('',*,*,#4807,.F.);
#6291=ORIENTED_EDGE('',*,*,#4808,.T.);
#6292=ORIENTED_EDGE('',*,*,#4789,.F.);
#6293=ORIENTED_EDGE('',*,*,#4808,.F.);
#6294=ORIENTED_EDGE('',*,*,#4809,.T.);
#6295=ORIENTED_EDGE('',*,*,#4810,.T.);
#6296=ORIENTED_EDGE('',*,*,#4811,.T.);
#6297=ORIENTED_EDGE('',*,*,#4810,.F.);
#6298=ORIENTED_EDGE('',*,*,#4809,.F.);
#6299=ORIENTED_EDGE('',*,*,#4812,.T.);
#6300=ORIENTED_EDGE('',*,*,#4813,.F.);
#6301=ORIENTED_EDGE('',*,*,#4814,.F.);
#6302=ORIENTED_EDGE('',*,*,#4815,.F.);
#6303=ORIENTED_EDGE('',*,*,#4816,.F.);
#6304=ORIENTED_EDGE('',*,*,#4817,.F.);
#6305=ORIENTED_EDGE('',*,*,#4818,.F.);
#6306=ORIENTED_EDGE('',*,*,#4819,.T.);
#6307=ORIENTED_EDGE('',*,*,#4820,.F.);
#6308=ORIENTED_EDGE('',*,*,#4821,.T.);
#6309=ORIENTED_EDGE('',*,*,#4822,.F.);
#6310=ORIENTED_EDGE('',*,*,#4823,.F.);
#6311=ORIENTED_EDGE('',*,*,#4824,.F.);
#6312=ORIENTED_EDGE('',*,*,#4825,.F.);
#6313=ORIENTED_EDGE('',*,*,#4826,.F.);
#6314=ORIENTED_EDGE('',*,*,#4827,.F.);
#6315=ORIENTED_EDGE('',*,*,#4828,.F.);
#6316=ORIENTED_EDGE('',*,*,#4829,.T.);
#6317=ORIENTED_EDGE('',*,*,#4830,.F.);
#6318=ORIENTED_EDGE('',*,*,#4831,.T.);
#6319=ORIENTED_EDGE('',*,*,#4832,.F.);
#6320=ORIENTED_EDGE('',*,*,#4833,.F.);
#6321=ORIENTED_EDGE('',*,*,#4834,.F.);
#6322=ORIENTED_EDGE('',*,*,#4835,.F.);
#6323=ORIENTED_EDGE('',*,*,#4836,.F.);
#6324=ORIENTED_EDGE('',*,*,#4837,.F.);
#6325=ORIENTED_EDGE('',*,*,#4838,.F.);
#6326=ORIENTED_EDGE('',*,*,#4839,.T.);
#6327=ORIENTED_EDGE('',*,*,#4840,.F.);
#6328=ORIENTED_EDGE('',*,*,#4841,.T.);
#6329=ORIENTED_EDGE('',*,*,#4842,.F.);
#6330=ORIENTED_EDGE('',*,*,#4843,.F.);
#6331=ORIENTED_EDGE('',*,*,#4844,.F.);
#6332=ORIENTED_EDGE('',*,*,#4845,.F.);
#6333=ORIENTED_EDGE('',*,*,#4846,.F.);
#6334=ORIENTED_EDGE('',*,*,#4847,.F.);
#6335=ORIENTED_EDGE('',*,*,#4848,.F.);
#6336=ORIENTED_EDGE('',*,*,#4849,.T.);
#6337=ORIENTED_EDGE('',*,*,#4850,.F.);
#6338=ORIENTED_EDGE('',*,*,#4851,.T.);
#6339=ORIENTED_EDGE('',*,*,#4852,.F.);
#6340=ORIENTED_EDGE('',*,*,#4853,.F.);
#6341=ORIENTED_EDGE('',*,*,#4812,.F.);
#6342=ORIENTED_EDGE('',*,*,#4854,.F.);
#6343=ORIENTED_EDGE('',*,*,#4811,.F.);
#6344=ORIENTED_EDGE('',*,*,#4844,.T.);
#6345=ORIENTED_EDGE('',*,*,#4855,.T.);
#6346=ORIENTED_EDGE('',*,*,#4856,.T.);
#6347=ORIENTED_EDGE('',*,*,#4857,.T.);
#6348=ORIENTED_EDGE('',*,*,#4856,.F.);
#6349=ORIENTED_EDGE('',*,*,#4858,.T.);
#6350=ORIENTED_EDGE('',*,*,#4859,.F.);
#6351=ORIENTED_EDGE('',*,*,#4860,.T.);
#6352=ORIENTED_EDGE('',*,*,#4855,.F.);
#6353=ORIENTED_EDGE('',*,*,#4843,.T.);
#6354=ORIENTED_EDGE('',*,*,#4861,.F.);
#6355=ORIENTED_EDGE('',*,*,#4858,.F.);
#6356=ORIENTED_EDGE('',*,*,#4859,.T.);
#6357=ORIENTED_EDGE('',*,*,#4861,.T.);
#6358=ORIENTED_EDGE('',*,*,#4842,.T.);
#6359=ORIENTED_EDGE('',*,*,#4862,.T.);
#6360=ORIENTED_EDGE('',*,*,#4834,.T.);
#6361=ORIENTED_EDGE('',*,*,#4863,.T.);
#6362=ORIENTED_EDGE('',*,*,#4864,.T.);
#6363=ORIENTED_EDGE('',*,*,#4865,.T.);
#6364=ORIENTED_EDGE('',*,*,#4863,.F.);
#6365=ORIENTED_EDGE('',*,*,#4833,.T.);
#6366=ORIENTED_EDGE('',*,*,#4866,.F.);
#6367=ORIENTED_EDGE('',*,*,#4867,.F.);
#6368=ORIENTED_EDGE('',*,*,#4868,.T.);
#6369=ORIENTED_EDGE('',*,*,#4869,.T.);
#6370=ORIENTED_EDGE('',*,*,#4852,.T.);
#6371=ORIENTED_EDGE('',*,*,#4870,.T.);
#6372=ORIENTED_EDGE('',*,*,#4869,.F.);
#6373=ORIENTED_EDGE('',*,*,#4871,.F.);
#6374=ORIENTED_EDGE('',*,*,#4872,.F.);
#6375=ORIENTED_EDGE('',*,*,#4813,.T.);
#6376=ORIENTED_EDGE('',*,*,#4853,.T.);
#6377=ORIENTED_EDGE('',*,*,#4814,.T.);
#6378=ORIENTED_EDGE('',*,*,#4872,.T.);
#6379=ORIENTED_EDGE('',*,*,#4873,.T.);
#6380=ORIENTED_EDGE('',*,*,#4874,.T.);
#6381=ORIENTED_EDGE('',*,*,#4875,.T.);
#6382=ORIENTED_EDGE('',*,*,#4876,.T.);
#6383=ORIENTED_EDGE('',*,*,#4822,.T.);
#6384=ORIENTED_EDGE('',*,*,#4877,.T.);
#6385=ORIENTED_EDGE('',*,*,#4876,.F.);
#6386=ORIENTED_EDGE('',*,*,#4878,.F.);
#6387=ORIENTED_EDGE('',*,*,#4879,.F.);
#6388=ORIENTED_EDGE('',*,*,#4823,.T.);
#6389=ORIENTED_EDGE('',*,*,#4875,.F.);
#6390=ORIENTED_EDGE('',*,*,#4880,.T.);
#6391=ORIENTED_EDGE('',*,*,#4881,.F.);
#6392=ORIENTED_EDGE('',*,*,#4878,.T.);
#6393=ORIENTED_EDGE('',*,*,#4882,.T.);
#6394=ORIENTED_EDGE('',*,*,#4866,.T.);
#6395=ORIENTED_EDGE('',*,*,#4832,.T.);
#6396=ORIENTED_EDGE('',*,*,#4883,.T.);
#6397=ORIENTED_EDGE('',*,*,#4864,.F.);
#6398=ORIENTED_EDGE('',*,*,#4867,.T.);
#6399=ORIENTED_EDGE('',*,*,#4882,.F.);
#6400=ORIENTED_EDGE('',*,*,#4884,.T.);
#6401=ORIENTED_EDGE('',*,*,#4824,.T.);
#6402=ORIENTED_EDGE('',*,*,#4879,.T.);
#6403=ORIENTED_EDGE('',*,*,#4881,.T.);
#6404=ORIENTED_EDGE('',*,*,#4885,.T.);
#6405=ORIENTED_EDGE('',*,*,#4885,.F.);
#6406=ORIENTED_EDGE('',*,*,#4886,.F.);
#6407=ORIENTED_EDGE('',*,*,#4887,.F.);
#6408=ORIENTED_EDGE('',*,*,#4825,.T.);
#6409=ORIENTED_EDGE('',*,*,#4836,.T.);
#6410=ORIENTED_EDGE('',*,*,#4888,.T.);
#6411=ORIENTED_EDGE('',*,*,#4889,.T.);
#6412=ORIENTED_EDGE('',*,*,#4890,.T.);
#6413=ORIENTED_EDGE('',*,*,#4891,.T.);
#6414=ORIENTED_EDGE('',*,*,#4890,.F.);
#6415=ORIENTED_EDGE('',*,*,#4892,.F.);
#6416=ORIENTED_EDGE('',*,*,#4893,.F.);
#6417=ORIENTED_EDGE('',*,*,#4799,.T.);
#6418=ORIENTED_EDGE('',*,*,#4889,.F.);
#6419=ORIENTED_EDGE('',*,*,#4894,.T.);
#6420=ORIENTED_EDGE('',*,*,#4895,.F.);
#6421=ORIENTED_EDGE('',*,*,#4892,.T.);
#6422=ORIENTED_EDGE('',*,*,#4896,.T.);
#6423=ORIENTED_EDGE('',*,*,#4897,.T.);
#6424=ORIENTED_EDGE('',*,*,#4840,.T.);
#6425=ORIENTED_EDGE('',*,*,#4898,.T.);
#6426=ORIENTED_EDGE('',*,*,#4899,.T.);
#6427=ORIENTED_EDGE('',*,*,#4896,.F.);
#6428=ORIENTED_EDGE('',*,*,#4900,.T.);
#6429=ORIENTED_EDGE('',*,*,#4901,.F.);
#6430=ORIENTED_EDGE('',*,*,#4902,.T.);
#6431=ORIENTED_EDGE('',*,*,#4899,.F.);
#6432=ORIENTED_EDGE('',*,*,#4795,.T.);
#6433=ORIENTED_EDGE('',*,*,#4903,.F.);
#6434=ORIENTED_EDGE('',*,*,#4900,.F.);
#6435=ORIENTED_EDGE('',*,*,#4846,.T.);
#6436=ORIENTED_EDGE('',*,*,#4904,.T.);
#6437=ORIENTED_EDGE('',*,*,#4901,.T.);
#6438=ORIENTED_EDGE('',*,*,#4903,.T.);
#6439=ORIENTED_EDGE('',*,*,#4905,.T.);
#6440=ORIENTED_EDGE('',*,*,#4857,.F.);
#6441=ORIENTED_EDGE('',*,*,#4906,.F.);
#6442=ORIENTED_EDGE('',*,*,#4904,.F.);
#6443=ORIENTED_EDGE('',*,*,#4845,.T.);
#6444=ORIENTED_EDGE('',*,*,#4907,.T.);
#6445=ORIENTED_EDGE('',*,*,#4908,.T.);
#6446=ORIENTED_EDGE('',*,*,#4850,.T.);
#6447=ORIENTED_EDGE('',*,*,#4909,.T.);
#6448=ORIENTED_EDGE('',*,*,#4910,.T.);
#6449=ORIENTED_EDGE('',*,*,#4907,.F.);
#6450=ORIENTED_EDGE('',*,*,#4911,.T.);
#6451=ORIENTED_EDGE('',*,*,#4912,.F.);
#6452=ORIENTED_EDGE('',*,*,#4913,.T.);
#6453=ORIENTED_EDGE('',*,*,#4910,.F.);
#6454=ORIENTED_EDGE('',*,*,#4791,.T.);
#6455=ORIENTED_EDGE('',*,*,#4807,.T.);
#6456=ORIENTED_EDGE('',*,*,#4914,.F.);
#6457=ORIENTED_EDGE('',*,*,#4911,.F.);
#6458=ORIENTED_EDGE('',*,*,#4816,.T.);
#6459=ORIENTED_EDGE('',*,*,#4915,.T.);
#6460=ORIENTED_EDGE('',*,*,#4912,.T.);
#6461=ORIENTED_EDGE('',*,*,#4914,.T.);
#6462=ORIENTED_EDGE('',*,*,#4916,.T.);
#6463=ORIENTED_EDGE('',*,*,#4874,.F.);
#6464=ORIENTED_EDGE('',*,*,#4917,.F.);
#6465=ORIENTED_EDGE('',*,*,#4915,.F.);
#6466=ORIENTED_EDGE('',*,*,#4815,.T.);
#6467=ORIENTED_EDGE('',*,*,#4918,.T.);
#6468=ORIENTED_EDGE('',*,*,#4919,.T.);
#6469=ORIENTED_EDGE('',*,*,#4820,.T.);
#6470=ORIENTED_EDGE('',*,*,#4920,.T.);
#6471=ORIENTED_EDGE('',*,*,#4921,.T.);
#6472=ORIENTED_EDGE('',*,*,#4918,.F.);
#6473=ORIENTED_EDGE('',*,*,#4922,.T.);
#6474=ORIENTED_EDGE('',*,*,#4923,.F.);
#6475=ORIENTED_EDGE('',*,*,#4924,.T.);
#6476=ORIENTED_EDGE('',*,*,#4921,.F.);
#6477=ORIENTED_EDGE('',*,*,#4803,.T.);
#6478=ORIENTED_EDGE('',*,*,#4925,.F.);
#6479=ORIENTED_EDGE('',*,*,#4922,.F.);
#6480=ORIENTED_EDGE('',*,*,#4895,.T.);
#6481=ORIENTED_EDGE('',*,*,#4926,.T.);
#6482=ORIENTED_EDGE('',*,*,#4830,.T.);
#6483=ORIENTED_EDGE('',*,*,#4927,.T.);
#6484=ORIENTED_EDGE('',*,*,#4893,.T.);
#6485=ORIENTED_EDGE('',*,*,#4826,.T.);
#6486=ORIENTED_EDGE('',*,*,#4887,.T.);
#6487=ORIENTED_EDGE('',*,*,#4923,.T.);
#6488=ORIENTED_EDGE('',*,*,#4925,.T.);
#6489=ORIENTED_EDGE('',*,*,#4928,.T.);
#6490=ORIENTED_EDGE('',*,*,#4929,.F.);
#6491=ORIENTED_EDGE('',*,*,#4796,.T.);
#6492=ORIENTED_EDGE('',*,*,#4898,.F.);
#6493=ORIENTED_EDGE('',*,*,#4839,.F.);
#6494=ORIENTED_EDGE('',*,*,#4930,.F.);
#6495=ORIENTED_EDGE('',*,*,#4847,.T.);
#6496=ORIENTED_EDGE('',*,*,#4905,.F.);
#6497=ORIENTED_EDGE('',*,*,#4794,.F.);
#6498=ORIENTED_EDGE('',*,*,#4931,.F.);
#6499=ORIENTED_EDGE('',*,*,#4800,.T.);
#6500=ORIENTED_EDGE('',*,*,#4927,.F.);
#6501=ORIENTED_EDGE('',*,*,#4829,.F.);
#6502=ORIENTED_EDGE('',*,*,#4932,.F.);
#6503=ORIENTED_EDGE('',*,*,#4837,.T.);
#6504=ORIENTED_EDGE('',*,*,#4891,.F.);
#6505=ORIENTED_EDGE('',*,*,#4798,.F.);
#6506=ORIENTED_EDGE('',*,*,#4933,.F.);
#6507=ORIENTED_EDGE('',*,*,#4792,.T.);
#6508=ORIENTED_EDGE('',*,*,#4909,.F.);
#6509=ORIENTED_EDGE('',*,*,#4849,.F.);
#6510=ORIENTED_EDGE('',*,*,#4934,.F.);
#6511=ORIENTED_EDGE('',*,*,#4817,.T.);
#6512=ORIENTED_EDGE('',*,*,#4916,.F.);
#6513=ORIENTED_EDGE('',*,*,#4806,.F.);
#6514=ORIENTED_EDGE('',*,*,#4935,.F.);
#6515=ORIENTED_EDGE('',*,*,#4804,.T.);
#6516=ORIENTED_EDGE('',*,*,#4920,.F.);
#6517=ORIENTED_EDGE('',*,*,#4819,.F.);
#6518=ORIENTED_EDGE('',*,*,#4936,.F.);
#6519=ORIENTED_EDGE('',*,*,#4827,.T.);
#6520=ORIENTED_EDGE('',*,*,#4928,.F.);
#6521=ORIENTED_EDGE('',*,*,#4802,.F.);
#6522=ORIENTED_EDGE('',*,*,#4932,.T.);
#6523=ORIENTED_EDGE('',*,*,#4797,.T.);
#6524=ORIENTED_EDGE('',*,*,#4929,.T.);
#6525=ORIENTED_EDGE('',*,*,#4838,.T.);
#6526=ORIENTED_EDGE('',*,*,#4936,.T.);
#6527=ORIENTED_EDGE('',*,*,#4801,.T.);
#6528=ORIENTED_EDGE('',*,*,#4931,.T.);
#6529=ORIENTED_EDGE('',*,*,#4828,.T.);
#6530=ORIENTED_EDGE('',*,*,#4930,.T.);
#6531=ORIENTED_EDGE('',*,*,#4793,.T.);
#6532=ORIENTED_EDGE('',*,*,#4933,.T.);
#6533=ORIENTED_EDGE('',*,*,#4848,.T.);
#6534=ORIENTED_EDGE('',*,*,#4934,.T.);
#6535=ORIENTED_EDGE('',*,*,#4805,.T.);
#6536=ORIENTED_EDGE('',*,*,#4935,.T.);
#6537=ORIENTED_EDGE('',*,*,#4818,.T.);
#6538=ORIENTED_EDGE('',*,*,#4790,.F.);
#6539=ORIENTED_EDGE('',*,*,#4937,.T.);
#6540=ORIENTED_EDGE('',*,*,#4854,.T.);
#6541=ORIENTED_EDGE('',*,*,#4937,.F.);
#6542=ORIENTED_EDGE('',*,*,#4865,.F.);
#6543=ORIENTED_EDGE('',*,*,#4938,.F.);
#6544=ORIENTED_EDGE('',*,*,#4888,.F.);
#6545=ORIENTED_EDGE('',*,*,#4835,.T.);
#6546=ORIENTED_EDGE('',*,*,#4884,.F.);
#6547=ORIENTED_EDGE('',*,*,#4939,.F.);
#6548=ORIENTED_EDGE('',*,*,#4894,.F.);
#6549=ORIENTED_EDGE('',*,*,#4938,.T.);
#6550=ORIENTED_EDGE('',*,*,#4883,.F.);
#6551=ORIENTED_EDGE('',*,*,#4831,.F.);
#6552=ORIENTED_EDGE('',*,*,#4926,.F.);
#6553=ORIENTED_EDGE('',*,*,#4939,.T.);
#6554=ORIENTED_EDGE('',*,*,#4868,.F.);
#6555=ORIENTED_EDGE('',*,*,#4940,.T.);
#6556=ORIENTED_EDGE('',*,*,#4873,.F.);
#6557=ORIENTED_EDGE('',*,*,#4871,.T.);
#6558=ORIENTED_EDGE('',*,*,#4940,.F.);
#6559=ORIENTED_EDGE('',*,*,#4941,.F.);
#6560=ORIENTED_EDGE('',*,*,#4913,.F.);
#6561=ORIENTED_EDGE('',*,*,#4917,.T.);
#6562=ORIENTED_EDGE('',*,*,#4870,.F.);
#6563=ORIENTED_EDGE('',*,*,#4851,.F.);
#6564=ORIENTED_EDGE('',*,*,#4908,.F.);
#6565=ORIENTED_EDGE('',*,*,#4941,.T.);
#6566=ORIENTED_EDGE('',*,*,#4880,.F.);
#6567=ORIENTED_EDGE('',*,*,#4942,.F.);
#6568=ORIENTED_EDGE('',*,*,#4924,.F.);
#6569=ORIENTED_EDGE('',*,*,#4886,.T.);
#6570=ORIENTED_EDGE('',*,*,#4877,.F.);
#6571=ORIENTED_EDGE('',*,*,#4821,.F.);
#6572=ORIENTED_EDGE('',*,*,#4919,.F.);
#6573=ORIENTED_EDGE('',*,*,#4942,.T.);
#6574=ORIENTED_EDGE('',*,*,#4860,.F.);
#6575=ORIENTED_EDGE('',*,*,#4943,.F.);
#6576=ORIENTED_EDGE('',*,*,#4902,.F.);
#6577=ORIENTED_EDGE('',*,*,#4906,.T.);
#6578=ORIENTED_EDGE('',*,*,#4862,.F.);
#6579=ORIENTED_EDGE('',*,*,#4841,.F.);
#6580=ORIENTED_EDGE('',*,*,#4897,.F.);
#6581=ORIENTED_EDGE('',*,*,#4943,.T.);
#9151=CYLINDRICAL_SURFACE('',#10146,0.00245);
#9152=CYLINDRICAL_SURFACE('',#10160,0.002);
#9153=CYLINDRICAL_SURFACE('',#10253,0.00345);
#9154=CYLINDRICAL_SURFACE('',#10255,0.00285);
#9155=CYLINDRICAL_SURFACE('',#10259,0.00285);
#9156=CYLINDRICAL_SURFACE('',#10261,0.00285);
#9157=CYLINDRICAL_SURFACE('',#10263,0.00285);
#9337=ADVANCED_FACE('',(#1115),#771,.F.);
#9338=ADVANCED_FACE('',(#1116,#710),#866,.T.);
#9339=ADVANCED_FACE('',(#1117),#9151,.T.);
#9340=ADVANCED_FACE('',(#1118),#772,.T.);
#9341=ADVANCED_FACE('',(#1119),#9152,.F.);
#9342=ADVANCED_FACE('',(#1120,#711),#867,.F.);
#9343=ADVANCED_FACE('',(#1121),#868,.T.);
#9344=ADVANCED_FACE('',(#1122),#605,.T.);
#9345=ADVANCED_FACE('',(#1123),#869,.T.);
#9346=ADVANCED_FACE('',(#1124),#870,.T.);
#9347=ADVANCED_FACE('',(#1125),#871,.T.);
#9348=ADVANCED_FACE('',(#1126),#872,.T.);
#9349=ADVANCED_FACE('',(#1127),#873,.T.);
#9350=ADVANCED_FACE('',(#1128),#874,.T.);
#9351=ADVANCED_FACE('',(#1129),#875,.T.);
#9352=ADVANCED_FACE('',(#1130),#876,.T.);
#9353=ADVANCED_FACE('',(#1131),#877,.T.);
#9354=ADVANCED_FACE('',(#1132),#606,.T.);
#9355=ADVANCED_FACE('',(#1133),#878,.T.);
#9356=ADVANCED_FACE('',(#1134),#607,.T.);
#9357=ADVANCED_FACE('',(#1135),#879,.T.);
#9358=ADVANCED_FACE('',(#1136),#880,.T.);
#9359=ADVANCED_FACE('',(#1137),#881,.T.);
#9360=ADVANCED_FACE('',(#1138),#882,.F.);
#9361=ADVANCED_FACE('',(#1139),#608,.T.);
#9362=ADVANCED_FACE('',(#1140),#883,.T.);
#9363=ADVANCED_FACE('',(#1141),#609,.T.);
#9364=ADVANCED_FACE('',(#1142),#884,.F.);
#9365=ADVANCED_FACE('',(#1143),#885,.T.);
#9366=ADVANCED_FACE('',(#1144),#886,.T.);
#9367=ADVANCED_FACE('',(#1145),#887,.T.);
#9368=ADVANCED_FACE('',(#1146),#610,.T.);
#9369=ADVANCED_FACE('',(#1147),#888,.F.);
#9370=ADVANCED_FACE('',(#1148),#889,.T.);
#9371=ADVANCED_FACE('',(#1149),#890,.T.);
#9372=ADVANCED_FACE('',(#1150),#891,.T.);
#9373=ADVANCED_FACE('',(#1151),#611,.T.);
#9374=ADVANCED_FACE('',(#1152),#892,.F.);
#9375=ADVANCED_FACE('',(#1153),#893,.T.);
#9376=ADVANCED_FACE('',(#1154),#894,.T.);
#9377=ADVANCED_FACE('',(#1155),#895,.T.);
#9378=ADVANCED_FACE('',(#1156),#896,.T.);
#9379=ADVANCED_FACE('',(#1157),#897,.T.);
#9380=ADVANCED_FACE('',(#1158),#898,.T.);
#9381=ADVANCED_FACE('',(#1159),#899,.T.);
#9382=ADVANCED_FACE('',(#1160),#900,.T.);
#9383=ADVANCED_FACE('',(#1161),#901,.T.);
#9384=ADVANCED_FACE('',(#1162),#902,.T.);
#9385=ADVANCED_FACE('',(#1163),#903,.T.);
#9386=ADVANCED_FACE('',(#1164),#904,.T.);
#9387=ADVANCED_FACE('',(#1165),#905,.T.);
#9388=ADVANCED_FACE('',(#1166),#906,.T.);
#9389=ADVANCED_FACE('',(#1167),#9153,.T.);
#9390=ADVANCED_FACE('',(#1168),#907,.T.);
#9391=ADVANCED_FACE('',(#1169),#9154,.T.);
#9392=ADVANCED_FACE('',(#1170),#908,.T.);
#9393=ADVANCED_FACE('',(#1171),#612,.T.);
#9394=ADVANCED_FACE('',(#1172),#9155,.T.);
#9395=ADVANCED_FACE('',(#1173),#909,.T.);
#9396=ADVANCED_FACE('',(#1174),#9156,.T.);
#9397=ADVANCED_FACE('',(#1175),#910,.T.);
#9398=ADVANCED_FACE('',(#1176),#9157,.T.);
#9399=ADVANCED_FACE('',(#1177),#911,.T.);
#9868=CLOSED_SHELL('',(#9337,#9338,#9339,#9340,#9341,#9342,#9343,#9344,
#9345,#9346,#9347,#9348,#9349,#9350,#9351,#9352,#9353,#9354,#9355,#9356,
#9357,#9358,#9359,#9360,#9361,#9362,#9363,#9364,#9365,#9366,#9367,#9368,
#9369,#9370,#9371,#9372,#9373,#9374,#9375,#9376,#9377,#9378,#9379,#9380,
#9381,#9382,#9383,#9384,#9385,#9386,#9387,#9388,#9389,#9390,#9391,#9392,
#9393,#9394,#9395,#9396,#9397,#9398,#9399));
#10139=AXIS2_PLACEMENT_3D('',#13523,#11106,#11107);
#10140=AXIS2_PLACEMENT_3D('',#13524,#11108,#11109);
#10141=AXIS2_PLACEMENT_3D('',#13526,#11110,#11111);
#10142=AXIS2_PLACEMENT_3D('',#13528,#11112,#11113);
#10143=AXIS2_PLACEMENT_3D('',#13529,#11114,#11115);
#10144=AXIS2_PLACEMENT_3D('',#13530,#11116,#11117);
#10145=AXIS2_PLACEMENT_3D('',#13532,#11118,#11119);
#10146=AXIS2_PLACEMENT_3D('',#13533,#11120,#11121);
#10147=AXIS2_PLACEMENT_3D('',#13536,#11122,#11123);
#10148=AXIS2_PLACEMENT_3D('',#13540,#11125,#11126);
#10149=AXIS2_PLACEMENT_3D('',#13544,#11128,#11129);
#10150=AXIS2_PLACEMENT_3D('',#13548,#11131,#11132);
#10151=AXIS2_PLACEMENT_3D('',#13552,#11134,#11135);
#10152=AXIS2_PLACEMENT_3D('',#13556,#11137,#11138);
#10153=AXIS2_PLACEMENT_3D('',#13560,#11140,#11141);
#10154=AXIS2_PLACEMENT_3D('',#13564,#11143,#11144);
#10155=AXIS2_PLACEMENT_3D('',#13567,#11146,#11147);
#10156=AXIS2_PLACEMENT_3D('',#13569,#11149,#11150);
#10157=AXIS2_PLACEMENT_3D('',#13571,#11151,#11152);
#10158=AXIS2_PLACEMENT_3D('',#13573,#11153,#11154);
#10159=AXIS2_PLACEMENT_3D('',#13574,#11155,#11156);
#10160=AXIS2_PLACEMENT_3D('',#13575,#11157,#11158);
#10161=AXIS2_PLACEMENT_3D('',#13579,#11160,#11161);
#10162=AXIS2_PLACEMENT_3D('',#13581,#11162,#11163);
#10163=AXIS2_PLACEMENT_3D('',#13585,#11165,#11166);
#10164=AXIS2_PLACEMENT_3D('',#13589,#11168,#11169);
#10165=AXIS2_PLACEMENT_3D('',#13593,#11171,#11172);
#10166=AXIS2_PLACEMENT_3D('',#13597,#11174,#11175);
#10167=AXIS2_PLACEMENT_3D('',#13599,#11176,#11177);
#10168=AXIS2_PLACEMENT_3D('',#13601,#11178,#11179);
#10169=AXIS2_PLACEMENT_3D('',#13605,#11181,#11182);
#10170=AXIS2_PLACEMENT_3D('',#13609,#11184,#11185);
#10171=AXIS2_PLACEMENT_3D('',#13613,#11187,#11188);
#10172=AXIS2_PLACEMENT_3D('',#13617,#11190,#11191);
#10173=AXIS2_PLACEMENT_3D('',#13619,#11192,#11193);
#10174=AXIS2_PLACEMENT_3D('',#13621,#11194,#11195);
#10175=AXIS2_PLACEMENT_3D('',#13625,#11197,#11198);
#10176=AXIS2_PLACEMENT_3D('',#13629,#11200,#11201);
#10177=AXIS2_PLACEMENT_3D('',#13633,#11203,#11204);
#10178=AXIS2_PLACEMENT_3D('',#13637,#11206,#11207);
#10179=AXIS2_PLACEMENT_3D('',#13639,#11208,#11209);
#10180=AXIS2_PLACEMENT_3D('',#13641,#11210,#11211);
#10181=AXIS2_PLACEMENT_3D('',#13645,#11213,#11214);
#10182=AXIS2_PLACEMENT_3D('',#13649,#11216,#11217);
#10183=AXIS2_PLACEMENT_3D('',#13653,#11219,#11220);
#10184=AXIS2_PLACEMENT_3D('',#13657,#11222,#11223);
#10185=AXIS2_PLACEMENT_3D('',#13658,#11224,#11225);
#10186=AXIS2_PLACEMENT_3D('',#13659,#11226,#11227);
#10187=AXIS2_PLACEMENT_3D('',#13661,#11228,#11229);
#10188=AXIS2_PLACEMENT_3D('',#13662,#11230,#11231);
#10189=AXIS2_PLACEMENT_3D('',#13670,#11234,#11235);
#10190=AXIS2_PLACEMENT_3D('',#13672,#11236,#11237);
#10191=AXIS2_PLACEMENT_3D('',#13677,#11238,#11239);
#10192=AXIS2_PLACEMENT_3D('',#13678,#11240,#11241);
#10193=AXIS2_PLACEMENT_3D('',#13680,#11243,#11244);
#10194=AXIS2_PLACEMENT_3D('',#13682,#11246,#11247);
#10195=AXIS2_PLACEMENT_3D('',#13690,#11250,#11251);
#10196=AXIS2_PLACEMENT_3D('',#13693,#11253,#11254);
#10197=AXIS2_PLACEMENT_3D('',#13694,#11255,#11256);
#10198=AXIS2_PLACEMENT_3D('',#13702,#11259,#11260);
#10199=AXIS2_PLACEMENT_3D('',#13704,#11261,#11262);
#10200=AXIS2_PLACEMENT_3D('',#13706,#11264,#11265);
#10201=AXIS2_PLACEMENT_3D('',#13712,#11267,#11268);
#10202=AXIS2_PLACEMENT_3D('',#13720,#11271,#11272);
#10203=AXIS2_PLACEMENT_3D('',#13722,#11273,#11274);
#10204=AXIS2_PLACEMENT_3D('',#13724,#11276,#11277);
#10205=AXIS2_PLACEMENT_3D('',#13726,#11278,#11279);
#10206=AXIS2_PLACEMENT_3D('',#13730,#11280,#11281);
#10207=AXIS2_PLACEMENT_3D('',#13736,#11283,#11284);
#10208=AXIS2_PLACEMENT_3D('',#13737,#11285,#11286);
#10209=AXIS2_PLACEMENT_3D('',#13738,#11287,#11288);
#10210=AXIS2_PLACEMENT_3D('',#13740,#11290,#11291);
#10211=AXIS2_PLACEMENT_3D('',#13744,#11294,#11295);
#10212=AXIS2_PLACEMENT_3D('',#13748,#11297,#11298);
#10213=AXIS2_PLACEMENT_3D('',#13751,#11301,#11302);
#10214=AXIS2_PLACEMENT_3D('',#13753,#11303,#11304);
#10215=AXIS2_PLACEMENT_3D('',#13755,#11306,#11307);
#10216=AXIS2_PLACEMENT_3D('',#13757,#11308,#11309);
#10217=AXIS2_PLACEMENT_3D('',#13758,#11310,#11311);
#10218=AXIS2_PLACEMENT_3D('',#13759,#11312,#11313);
#10219=AXIS2_PLACEMENT_3D('',#13768,#11317,#11318);
#10220=AXIS2_PLACEMENT_3D('',#13770,#11319,#11320);
#10221=AXIS2_PLACEMENT_3D('',#13775,#11321,#11322);
#10222=AXIS2_PLACEMENT_3D('',#13776,#11323,#11324);
#10223=AXIS2_PLACEMENT_3D('',#13778,#11326,#11327);
#10224=AXIS2_PLACEMENT_3D('',#13781,#11330,#11331);
#10225=AXIS2_PLACEMENT_3D('',#13783,#11333,#11334);
#10226=AXIS2_PLACEMENT_3D('',#13786,#11335,#11336);
#10227=AXIS2_PLACEMENT_3D('',#13790,#11340,#11341);
#10228=AXIS2_PLACEMENT_3D('',#13792,#11342,#11343);
#10229=AXIS2_PLACEMENT_3D('',#13794,#11344,#11345);
#10230=AXIS2_PLACEMENT_3D('',#13795,#11346,#11347);
#10231=AXIS2_PLACEMENT_3D('',#13796,#11348,#11349);
#10232=AXIS2_PLACEMENT_3D('',#13798,#11351,#11352);
#10233=AXIS2_PLACEMENT_3D('',#13801,#11355,#11356);
#10234=AXIS2_PLACEMENT_3D('',#13803,#11358,#11359);
#10235=AXIS2_PLACEMENT_3D('',#13812,#11363,#11364);
#10236=AXIS2_PLACEMENT_3D('',#13814,#11365,#11366);
#10237=AXIS2_PLACEMENT_3D('',#13818,#11367,#11368);
#10238=AXIS2_PLACEMENT_3D('',#13819,#11369,#11370);
#10239=AXIS2_PLACEMENT_3D('',#13821,#11372,#11373);
#10240=AXIS2_PLACEMENT_3D('',#13824,#11376,#11377);
#10241=AXIS2_PLACEMENT_3D('',#13826,#11379,#11380);
#10242=AXIS2_PLACEMENT_3D('',#13828,#11382,#11383);
#10243=AXIS2_PLACEMENT_3D('',#13830,#11385,#11386);
#10244=AXIS2_PLACEMENT_3D('',#13832,#11388,#11389);
#10245=AXIS2_PLACEMENT_3D('',#13834,#11391,#11392);
#10246=AXIS2_PLACEMENT_3D('',#13836,#11394,#11395);
#10247=AXIS2_PLACEMENT_3D('',#13838,#11397,#11398);
#10248=AXIS2_PLACEMENT_3D('',#13840,#11400,#11401);
#10249=AXIS2_PLACEMENT_3D('',#13842,#11403,#11404);
#10250=AXIS2_PLACEMENT_3D('',#13843,#11405,#11406);
#10251=AXIS2_PLACEMENT_3D('',#13844,#11407,#11408);
#10252=AXIS2_PLACEMENT_3D('',#13845,#11409,#11410);
#10253=AXIS2_PLACEMENT_3D('',#13846,#11411,#11412);
#10254=AXIS2_PLACEMENT_3D('',#13848,#11414,#11415);
#10255=AXIS2_PLACEMENT_3D('',#13850,#11417,#11418);
#10256=AXIS2_PLACEMENT_3D('',#13852,#11420,#11421);
#10257=AXIS2_PLACEMENT_3D('',#13853,#11422,#11423);
#10258=AXIS2_PLACEMENT_3D('',#13854,#11424,#11425);
#10259=AXIS2_PLACEMENT_3D('',#13855,#11426,#11427);
#10260=AXIS2_PLACEMENT_3D('',#13857,#11429,#11430);
#10261=AXIS2_PLACEMENT_3D('',#13858,#11431,#11432);
#10262=AXIS2_PLACEMENT_3D('',#13860,#11434,#11435);
#10263=AXIS2_PLACEMENT_3D('',#13861,#11436,#11437);
#10264=AXIS2_PLACEMENT_3D('',#13863,#11439,#11440);
#11106=DIRECTION('axis',(0.,0.,1.));
#11107=DIRECTION('refdir',(1.,0.,0.));
#11108=DIRECTION('center_axis',(0.,1.,1.04083408558608E-15));
#11109=DIRECTION('ref_axis',(-1.,0.,0.));
#11110=DIRECTION('center_axis',(0.,-1.,-1.04083408558608E-15));
#11111=DIRECTION('ref_axis',(-0.387755102042543,-9.5940175792169E-16,0.921762431887944));
#11112=DIRECTION('center_axis',(0.,-1.04083408558608E-15,1.));
#11113=DIRECTION('ref_axis',(1.,0.,0.));
#11114=DIRECTION('center_axis',(0.,1.,1.04083408558608E-15));
#11115=DIRECTION('ref_axis',(-0.387755102042826,-9.59401757921566E-16,0.921762431887825));
#11116=DIRECTION('center_axis',(0.,-1.,-1.04083408558608E-15));
#11117=DIRECTION('ref_axis',(1.,0.,0.));
#11118=DIRECTION('center_axis',(0.,-1.,-1.04083408558608E-15));
#11119=DIRECTION('ref_axis',(1.,0.,0.));
#11120=DIRECTION('center_axis',(0.,-1.,-1.04083408558608E-15));
#11121=DIRECTION('ref_axis',(-1.,0.,0.));
#11122=DIRECTION('center_axis',(0.,-1.,-1.04083408558608E-15));
#11123=DIRECTION('ref_axis',(-1.,0.,0.));
#11124=DIRECTION('',(0.,-1.,-1.04083408558608E-15));
#11125=DIRECTION('center_axis',(0.,-1.,-1.04083408558608E-15));
#11126=DIRECTION('ref_axis',(-1.,0.,0.));
#11127=DIRECTION('',(0.,-1.,-1.04083408558608E-15));
#11128=DIRECTION('center_axis',(0.,-1.,-1.04083408558608E-15));
#11129=DIRECTION('ref_axis',(-1.,0.,0.));
#11130=DIRECTION('',(0.,-1.,-1.04083408558608E-15));
#11131=DIRECTION('center_axis',(0.,-1.,-1.04083408558608E-15));
#11132=DIRECTION('ref_axis',(-1.,0.,0.));
#11133=DIRECTION('',(0.,-1.,-1.04083408558608E-15));
#11134=DIRECTION('center_axis',(0.,-1.,-1.04083408558608E-15));
#11135=DIRECTION('ref_axis',(-1.,0.,0.));
#11136=DIRECTION('',(0.,-1.,-1.04083408558608E-15));
#11137=DIRECTION('center_axis',(0.,-1.,-1.04083408558608E-15));
#11138=DIRECTION('ref_axis',(-1.,0.,0.));
#11139=DIRECTION('',(0.,-1.,-1.04083408558608E-15));
#11140=DIRECTION('center_axis',(0.,-1.,-1.04083408558608E-15));
#11141=DIRECTION('ref_axis',(-1.,0.,0.));
#11142=DIRECTION('',(0.,-1.,-1.04083408558608E-15));
#11143=DIRECTION('center_axis',(0.,-1.,-1.04083408558608E-15));
#11144=DIRECTION('ref_axis',(-1.,0.,0.));
#11145=DIRECTION('',(0.,-1.,-1.04083408558608E-15));
#11146=DIRECTION('center_axis',(0.,-1.,-1.04083408558608E-15));
#11147=DIRECTION('ref_axis',(-1.,0.,0.));
#11148=DIRECTION('',(0.,1.,1.04083408558608E-15));
#11149=DIRECTION('center_axis',(0.,1.,1.04083408558608E-15));
#11150=DIRECTION('ref_axis',(-1.,0.,0.));
#11151=DIRECTION('center_axis',(0.,-1.,-1.04083408558608E-15));
#11152=DIRECTION('ref_axis',(1.,0.,0.));
#11153=DIRECTION('center_axis',(0.,1.04083408558608E-15,-1.));
#11154=DIRECTION('ref_axis',(1.,0.,0.));
#11155=DIRECTION('center_axis',(0.,1.,1.04083408558608E-15));
#11156=DIRECTION('ref_axis',(1.,0.,0.));
#11157=DIRECTION('center_axis',(0.,-1.,-1.04083408558608E-15));
#11158=DIRECTION('ref_axis',(-1.,0.,0.));
#11159=DIRECTION('',(0.,-1.,-1.04083408558608E-15));
#11160=DIRECTION('center_axis',(0.,1.,1.04083408558608E-15));
#11161=DIRECTION('ref_axis',(-1.,0.,0.));
#11162=DIRECTION('center_axis',(0.,0.083045479854119,-0.996545758244848));
#11163=DIRECTION('ref_axis',(0.,-0.996545758244848,-0.083045479854119));
#11164=DIRECTION('',(0.,-1.,-1.04083408558608E-15));
#11165=DIRECTION('center_axis',(0.,-0.196116135138937,-0.98058067569077));
#11166=DIRECTION('ref_axis',(0.,0.98058067569077,-0.196116135138937));
#11167=DIRECTION('',(0.,-1.,-1.04083408558608E-15));
#11168=DIRECTION('center_axis',(0.,1.,1.04083408558608E-15));
#11169=DIRECTION('ref_axis',(-1.,0.,0.));
#11170=DIRECTION('',(0.,-1.,-1.04083408558608E-15));
#11171=DIRECTION('center_axis',(-0.980580675690769,-0.196116135138938,-2.04124358186013E-16));
#11172=DIRECTION('ref_axis',(-0.196116135138938,0.980580675690769,1.02062179092598E-15));
#11173=DIRECTION('',(0.,-1.,-1.04083408558608E-15));
#11174=DIRECTION('center_axis',(-0.996545758244848,0.083045479854118,8.64365660860182E-17));
#11175=DIRECTION('ref_axis',(-0.083045479854118,-0.996545758244848,-1.03723879302746E-15));
#11176=DIRECTION('center_axis',(0.,1.,1.04083408558608E-15));
#11177=DIRECTION('ref_axis',(-1.,0.,0.));
#11178=DIRECTION('center_axis',(0.996545758244848,0.083045479854118,8.64365660860182E-17));
#11179=DIRECTION('ref_axis',(-0.083045479854118,0.996545758244848,1.03723879302746E-15));
#11180=DIRECTION('',(0.,-1.,-1.04083408558608E-15));
#11181=DIRECTION('center_axis',(0.980580675690769,-0.196116135138938,-2.04124358186013E-16));
#11182=DIRECTION('ref_axis',(-0.196116135138938,-0.980580675690769,-1.02062179092598E-15));
#11183=DIRECTION('',(0.,-1.,-1.04083408558608E-15));
#11184=DIRECTION('center_axis',(0.,1.,1.04083408558608E-15));
#11185=DIRECTION('ref_axis',(-1.,0.,0.));
#11186=DIRECTION('',(0.,-1.,-1.04083408558608E-15));
#11187=DIRECTION('center_axis',(0.,-0.196116135138937,-0.98058067569077));
#11188=DIRECTION('ref_axis',(0.,0.98058067569077,-0.196116135138937));
#11189=DIRECTION('',(0.,-1.,-1.04083408558608E-15));
#11190=DIRECTION('center_axis',(0.,0.083045479854119,-0.996545758244848));
#11191=DIRECTION('ref_axis',(0.,-0.996545758244848,-0.083045479854119));
#11192=DIRECTION('center_axis',(0.,1.,1.04083408558608E-15));
#11193=DIRECTION('ref_axis',(-1.,0.,0.));
#11194=DIRECTION('center_axis',(0.,0.083045479854117,0.996545758244848));
#11195=DIRECTION('ref_axis',(0.,0.996545758244848,-0.083045479854117));
#11196=DIRECTION('',(0.,-1.,-1.04083408558608E-15));
#11197=DIRECTION('center_axis',(0.,-0.196116135138939,0.980580675690769));
#11198=DIRECTION('ref_axis',(0.,-0.980580675690769,-0.196116135138939));
#11199=DIRECTION('',(0.,-1.,-1.04083408558608E-15));
#11200=DIRECTION('center_axis',(0.,1.,1.04083408558608E-15));
#11201=DIRECTION('ref_axis',(-1.,0.,0.));
#11202=DIRECTION('',(0.,-1.,-1.04083408558608E-15));
#11203=DIRECTION('center_axis',(0.980580675690769,-0.196116135138938,-2.04124358186013E-16));
#11204=DIRECTION('ref_axis',(-0.196116135138938,-0.980580675690769,-1.02062179092598E-15));
#11205=DIRECTION('',(0.,-1.,-1.04083408558608E-15));
#11206=DIRECTION('center_axis',(0.996545758244848,0.083045479854118,8.64365660860182E-17));
#11207=DIRECTION('ref_axis',(-0.083045479854118,0.996545758244848,1.03723879302746E-15));
#11208=DIRECTION('center_axis',(0.,1.,1.04083408558608E-15));
#11209=DIRECTION('ref_axis',(-1.,0.,0.));
#11210=DIRECTION('center_axis',(-0.996545758244848,0.083045479854118,8.64365660860182E-17));
#11211=DIRECTION('ref_axis',(-0.083045479854118,-0.996545758244848,-1.03723879302746E-15));
#11212=DIRECTION('',(0.,-1.,-1.04083408558608E-15));
#11213=DIRECTION('center_axis',(-0.980580675690769,-0.196116135138938,-2.04124358186013E-16));
#11214=DIRECTION('ref_axis',(-0.196116135138938,0.980580675690769,1.02062179092598E-15));
#11215=DIRECTION('',(0.,-1.,-1.04083408558608E-15));
#11216=DIRECTION('center_axis',(0.,1.,1.04083408558608E-15));
#11217=DIRECTION('ref_axis',(-1.,0.,0.));
#11218=DIRECTION('',(0.,-1.,-1.04083408558608E-15));
#11219=DIRECTION('center_axis',(0.,-0.196116135138939,0.980580675690769));
#11220=DIRECTION('ref_axis',(0.,-0.980580675690769,-0.196116135138939));
#11221=DIRECTION('',(0.,-1.,-1.04083408558608E-15));
#11222=DIRECTION('center_axis',(0.,0.083045479854117,0.996545758244848));
#11223=DIRECTION('ref_axis',(0.,0.996545758244848,-0.083045479854117));
#11224=DIRECTION('center_axis',(0.,1.,1.04083408558608E-15));
#11225=DIRECTION('ref_axis',(-1.,0.,0.));
#11226=DIRECTION('center_axis',(0.,-1.,-1.04083408558608E-15));
#11227=DIRECTION('ref_axis',(1.,0.,0.));
#11228=DIRECTION('center_axis',(0.,-1.,-1.04083408558608E-15));
#11229=DIRECTION('ref_axis',(1.,0.,0.));
#11230=DIRECTION('center_axis',(0.99654575824488,-0.08304547985374,-8.64365660856247E-17));
#11231=DIRECTION('ref_axis',(8.26770005765773E-33,1.04083408558608E-15,
-1.));
#11232=DIRECTION('',(0.,1.04083408558608E-15,-1.));
#11233=DIRECTION('',(0.,-1.04083408558608E-15,1.));
#11234=DIRECTION('center_axis',(0.,1.,1.04083408558608E-15));
#11235=DIRECTION('ref_axis',(-1.,0.,0.));
#11236=DIRECTION('center_axis',(0.,1.,1.04083408558608E-15));
#11237=DIRECTION('ref_axis',(-1.,0.,0.));
#11238=DIRECTION('center_axis',(0.,-1.,-1.04083408558608E-15));
#11239=DIRECTION('ref_axis',(-1.,0.,0.));
#11240=DIRECTION('center_axis',(0.,-1.,-1.04083408558608E-15));
#11241=DIRECTION('ref_axis',(1.,0.,0.));
#11242=DIRECTION('',(0.,-1.04083408558608E-15,1.));
#11243=DIRECTION('center_axis',(-0.99654575824488,-0.08304547985374,-8.64365660856247E-17));
#11244=DIRECTION('ref_axis',(8.26770005765773E-33,-1.04083408558608E-15,
1.));
#11245=DIRECTION('',(0.,1.04083408558608E-15,-1.));
#11246=DIRECTION('center_axis',(0.,-0.083045479853739,-0.99654575824488));
#11247=DIRECTION('ref_axis',(-1.,0.,0.));
#11248=DIRECTION('',(-1.,0.,0.));
#11249=DIRECTION('',(1.,0.,0.));
#11250=DIRECTION('center_axis',(0.,-1.,-1.04083408558608E-15));
#11251=DIRECTION('ref_axis',(1.,0.,0.));
#11252=DIRECTION('',(1.,0.,0.));
#11253=DIRECTION('center_axis',(0.,1.,1.04083408558608E-15));
#11254=DIRECTION('ref_axis',(-1.,0.,0.));
#11255=DIRECTION('center_axis',(0.,-0.083045479853739,-0.99654575824488));
#11256=DIRECTION('ref_axis',(-1.,0.,0.));
#11257=DIRECTION('',(-1.,0.,0.));
#11258=DIRECTION('',(1.,0.,0.));
#11259=DIRECTION('center_axis',(0.,-1.,-1.04083408558608E-15));
#11260=DIRECTION('ref_axis',(1.,0.,0.));
#11261=DIRECTION('center_axis',(0.,1.,1.04083408558608E-15));
#11262=DIRECTION('ref_axis',(1.,0.,0.));
#11263=DIRECTION('',(1.,0.,0.));
#11264=DIRECTION('center_axis',(0.,-0.083045479853741,0.99654575824488));
#11265=DIRECTION('ref_axis',(1.,0.,0.));
#11266=DIRECTION('',(-1.,0.,0.));
#11267=DIRECTION('center_axis',(0.99654575824488,-0.08304547985374,-8.64365660856247E-17));
#11268=DIRECTION('ref_axis',(8.26770005765773E-33,1.04083408558608E-15,
-1.));
#11269=DIRECTION('',(0.,1.04083408558608E-15,-1.));
#11270=DIRECTION('',(0.,-1.04083408558608E-15,1.));
#11271=DIRECTION('center_axis',(0.,-1.,-1.04083408558608E-15));
#11272=DIRECTION('ref_axis',(1.,0.,0.));
#11273=DIRECTION('center_axis',(0.,1.,1.04083408558608E-15));
#11274=DIRECTION('ref_axis',(-1.,0.,0.));
#11275=DIRECTION('',(0.,-1.04083408558608E-15,1.));
#11276=DIRECTION('center_axis',(0.,1.,1.04083408558608E-15));
#11277=DIRECTION('ref_axis',(-1.,0.,0.));
#11278=DIRECTION('center_axis',(0.,-1.,-1.04083408558608E-15));
#11279=DIRECTION('ref_axis',(-1.,0.,0.));
#11280=DIRECTION('center_axis',(0.,-0.083045479853741,0.99654575824488));
#11281=DIRECTION('ref_axis',(1.,0.,0.));
#11282=DIRECTION('',(-1.,0.,0.));
#11283=DIRECTION('center_axis',(0.,1.,1.04083408558608E-15));
#11284=DIRECTION('ref_axis',(-1.,0.,0.));
#11285=DIRECTION('center_axis',(0.,-1.,-1.04083408558608E-15));
#11286=DIRECTION('ref_axis',(-1.,0.,0.));
#11287=DIRECTION('center_axis',(-0.99654575824488,-0.08304547985374,-8.64365660856247E-17));
#11288=DIRECTION('ref_axis',(8.26770005765773E-33,-1.04083408558608E-15,
1.));
#11289=DIRECTION('',(0.,1.04083408558608E-15,-1.));
#11290=DIRECTION('center_axis',(-1.,0.,0.));
#11291=DIRECTION('ref_axis',(0.,-1.,-1.04083408558608E-15));
#11292=DIRECTION('',(0.,-1.,-1.04083408558608E-15));
#11293=DIRECTION('',(0.,-1.04083408558608E-15,1.));
#11294=DIRECTION('center_axis',(0.,0.196116135138185,-0.98058067569092));
#11295=DIRECTION('ref_axis',(0.,0.98058067569092,0.196116135138185));
#11296=DIRECTION('',(-1.,0.,0.));
#11297=DIRECTION('center_axis',(-2.93579933474955E-11,0.196116135154336,
-0.98058067568769));
#11298=DIRECTION('ref_axis',(-0.872297796013763,0.479479440345853,0.0958958881035005));
#11299=DIRECTION('',(1.,0.,0.));
#11300=DIRECTION('',(1.,0.,0.));
#11301=DIRECTION('center_axis',(0.,-1.,-1.04083408558608E-15));
#11302=DIRECTION('ref_axis',(1.,0.,0.));
#11303=DIRECTION('center_axis',(0.,-1.,-1.04083408558608E-15));
#11304=DIRECTION('ref_axis',(-1.,0.,0.));
#11305=DIRECTION('',(-1.,0.,0.));
#11306=DIRECTION('center_axis',(0.,-1.,-1.04083408558608E-15));
#11307=DIRECTION('ref_axis',(-1.,0.,0.));
#11308=DIRECTION('center_axis',(0.,1.,1.04083408558608E-15));
#11309=DIRECTION('ref_axis',(-1.,0.,0.));
#11310=DIRECTION('center_axis',(-2.93579933474955E-11,0.196116135154334,
0.98058067568769));
#11311=DIRECTION('ref_axis',(-0.871703578481421,0.480517420696057,-0.0961034841735403));
#11312=DIRECTION('center_axis',(-0.98058067569092,0.196116135138184,2.04124358185228E-16));
#11313=DIRECTION('ref_axis',(-0.196116135138184,-0.98058067569092,-1.02062179092614E-15));
#11314=DIRECTION('',(0.,-1.04083408558608E-15,1.));
#11315=DIRECTION('',(0.,1.04083408558608E-15,-1.));
#11316=DIRECTION('',(0.,1.04083408558608E-15,-1.));
#11317=DIRECTION('center_axis',(0.,-1.,-1.04083408558608E-15));
#11318=DIRECTION('ref_axis',(-1.,0.,0.));
#11319=DIRECTION('center_axis',(0.,-1.,-1.04083408558608E-15));
#11320=DIRECTION('ref_axis',(-1.,0.,0.));
#11321=DIRECTION('center_axis',(0.,1.,1.04083408558608E-15));
#11322=DIRECTION('ref_axis',(-1.,0.,0.));
#11323=DIRECTION('center_axis',(0.,-1.,-1.04083408558608E-15));
#11324=DIRECTION('ref_axis',(1.,0.,0.));
#11325=DIRECTION('',(0.,-1.04083408558608E-15,1.));
#11326=DIRECTION('center_axis',(0.98058067569092,0.196116135138184,2.04124358185228E-16));
#11327=DIRECTION('ref_axis',(1.87305315315727E-31,1.04083408558608E-15,
-1.));
#11328=DIRECTION('',(0.,1.04083408558608E-15,-1.));
#11329=DIRECTION('',(0.,-1.04083408558608E-15,1.));
#11330=DIRECTION('center_axis',(1.,0.,0.));
#11331=DIRECTION('ref_axis',(0.,-1.04083408558608E-15,1.));
#11332=DIRECTION('',(0.,-1.,-1.04083408558608E-15));
#11333=DIRECTION('center_axis',(0.,0.196116135138185,-0.98058067569092));
#11334=DIRECTION('ref_axis',(0.,0.98058067569092,0.196116135138185));
#11335=DIRECTION('center_axis',(2.93579933474955E-11,0.196116135154336,
-0.98058067568769));
#11336=DIRECTION('ref_axis',(0.871703578481421,0.480517420696057,0.0961034841735413));
#11337=DIRECTION('',(-1.,0.,0.));
#11338=DIRECTION('',(1.,0.,0.));
#11339=DIRECTION('',(1.,0.,0.));
#11340=DIRECTION('center_axis',(0.,-1.,-1.04083408558608E-15));
#11341=DIRECTION('ref_axis',(1.,0.,0.));
#11342=DIRECTION('center_axis',(0.,-1.,-1.04083408558608E-15));
#11343=DIRECTION('ref_axis',(1.,0.,0.));
#11344=DIRECTION('center_axis',(2.93579933474955E-11,0.196116135154334,
0.98058067568769));
#11345=DIRECTION('ref_axis',(0.872297796013763,0.479479440345853,-0.0958958881034995));
#11346=DIRECTION('center_axis',(0.,1.,1.04083408558608E-15));
#11347=DIRECTION('ref_axis',(1.,0.,0.));
#11348=DIRECTION('center_axis',(0.,-1.,-1.04083408558608E-15));
#11349=DIRECTION('ref_axis',(1.,0.,0.));
#11350=DIRECTION('',(-1.,0.,0.));
#11351=DIRECTION('center_axis',(0.,0.196116135138183,0.98058067569092));
#11352=DIRECTION('ref_axis',(-1.,0.,0.));
#11353=DIRECTION('',(1.,0.,0.));
#11354=DIRECTION('',(-1.,0.,0.));
#11355=DIRECTION('center_axis',(0.,-1.04083408558608E-15,1.));
#11356=DIRECTION('ref_axis',(1.,0.,0.));
#11357=DIRECTION('',(0.,-1.,-1.04083408558608E-15));
#11358=DIRECTION('center_axis',(0.98058067569092,0.196116135138184,2.04124358185228E-16));
#11359=DIRECTION('ref_axis',(1.87305315315727E-31,1.04083408558608E-15,
-1.));
#11360=DIRECTION('',(0.,1.04083408558608E-15,-1.));
#11361=DIRECTION('',(0.,-1.04083408558608E-15,1.));
#11362=DIRECTION('',(0.,-1.04083408558608E-15,1.));
#11363=DIRECTION('center_axis',(0.,-1.,-1.04083408558608E-15));
#11364=DIRECTION('ref_axis',(-1.,0.,0.));
#11365=DIRECTION('center_axis',(0.,-1.,-1.04083408558608E-15));
#11366=DIRECTION('ref_axis',(-1.,0.,0.));
#11367=DIRECTION('center_axis',(0.,1.,1.04083408558608E-15));
#11368=DIRECTION('ref_axis',(-1.,0.,0.));
#11369=DIRECTION('center_axis',(0.,-1.,-1.04083408558608E-15));
#11370=DIRECTION('ref_axis',(1.,0.,0.));
#11371=DIRECTION('',(0.,1.04083408558608E-15,-1.));
#11372=DIRECTION('center_axis',(0.,0.196116135138183,0.98058067569092));
#11373=DIRECTION('ref_axis',(-1.,0.,0.));
#11374=DIRECTION('',(1.,0.,0.));
#11375=DIRECTION('',(-1.,0.,0.));
#11376=DIRECTION('center_axis',(-0.98058067569092,0.196116135138184,2.04124358185228E-16));
#11377=DIRECTION('ref_axis',(-0.196116135138184,-0.98058067569092,-1.02062179092614E-15));
#11378=DIRECTION('',(0.,1.04083408558608E-15,-1.));
#11379=DIRECTION('center_axis',(-1.,0.,0.));
#11380=DIRECTION('ref_axis',(0.,-1.,-1.04083408558608E-15));
#11381=DIRECTION('',(0.,-1.04083408558608E-15,1.));
#11382=DIRECTION('center_axis',(1.,0.,0.));
#11383=DIRECTION('ref_axis',(0.,-1.04083408558608E-15,1.));
#11384=DIRECTION('',(0.,1.04083408558608E-15,-1.));
#11385=DIRECTION('center_axis',(0.,-1.04083408558608E-15,1.));
#11386=DIRECTION('ref_axis',(1.,0.,0.));
#11387=DIRECTION('',(1.,0.,0.));
#11388=DIRECTION('center_axis',(0.,1.04083408558608E-15,-1.));
#11389=DIRECTION('ref_axis',(0.,1.,1.04083408558608E-15));
#11390=DIRECTION('',(-1.,0.,0.));
#11391=DIRECTION('center_axis',(0.,1.04083408558608E-15,-1.));
#11392=DIRECTION('ref_axis',(0.,1.,1.04083408558608E-15));
#11393=DIRECTION('',(-1.,0.,0.));
#11394=DIRECTION('center_axis',(0.,-1.04083408558608E-15,1.));
#11395=DIRECTION('ref_axis',(1.,0.,0.));
#11396=DIRECTION('',(1.,0.,0.));
#11397=DIRECTION('center_axis',(1.,0.,0.));
#11398=DIRECTION('ref_axis',(0.,-1.04083408558608E-15,1.));
#11399=DIRECTION('',(0.,1.04083408558608E-15,-1.));
#11400=DIRECTION('center_axis',(-1.,0.,0.));
#11401=DIRECTION('ref_axis',(0.,-1.,-1.04083408558608E-15));
#11402=DIRECTION('',(0.,-1.04083408558608E-15,1.));
#11403=DIRECTION('center_axis',(0.,-1.,-1.04083408558608E-15));
#11404=DIRECTION('ref_axis',(1.,0.,0.));
#11405=DIRECTION('center_axis',(0.,-1.,-1.04083408558608E-15));
#11406=DIRECTION('ref_axis',(1.,0.,0.));
#11407=DIRECTION('center_axis',(0.,-1.,-1.04083408558608E-15));
#11408=DIRECTION('ref_axis',(1.,0.,0.));
#11409=DIRECTION('center_axis',(0.,-1.,-1.04083408558608E-15));
#11410=DIRECTION('ref_axis',(1.,0.,0.));
#11411=DIRECTION('center_axis',(0.,-1.,-1.04083408558608E-15));
#11412=DIRECTION('ref_axis',(1.,0.,0.));
#11413=DIRECTION('',(0.,1.,1.04083408558608E-15));
#11414=DIRECTION('center_axis',(0.,1.04083408558608E-15,-1.));
#11415=DIRECTION('ref_axis',(0.,1.,1.04083408558608E-15));
#11416=DIRECTION('',(0.,-1.,-1.04083408558608E-15));
#11417=DIRECTION('center_axis',(0.,-1.,-1.04083408558608E-15));
#11418=DIRECTION('ref_axis',(-1.,0.,0.));
#11419=DIRECTION('',(0.,-1.,-1.04083408558608E-15));
#11420=DIRECTION('center_axis',(0.,-1.04083408558608E-15,1.));
#11421=DIRECTION('ref_axis',(1.,0.,0.));
#11422=DIRECTION('center_axis',(0.,1.,1.04083408558608E-15));
#11423=DIRECTION('ref_axis',(1.,0.,0.));
#11424=DIRECTION('center_axis',(0.,-1.,-1.04083408558608E-15));
#11425=DIRECTION('ref_axis',(1.,0.,0.));
#11426=DIRECTION('center_axis',(0.,-1.,-1.04083408558608E-15));
#11427=DIRECTION('ref_axis',(1.,1.27465413135645E-31,-1.22464679914735E-16));
#11428=DIRECTION('',(0.,-1.,-1.04083408558608E-15));
#11429=DIRECTION('center_axis',(0.,1.04083408558608E-15,-1.));
#11430=DIRECTION('ref_axis',(0.,1.,1.04083408558608E-15));
#11431=DIRECTION('center_axis',(0.,-1.,-1.04083408558608E-15));
#11432=DIRECTION('ref_axis',(-1.,0.,0.));
#11433=DIRECTION('',(0.,-1.,-1.04083408558608E-15));
#11434=DIRECTION('center_axis',(1.,0.,0.));
#11435=DIRECTION('ref_axis',(0.,-1.04083408558608E-15,1.));
#11436=DIRECTION('center_axis',(0.,-1.,-1.04083408558608E-15));
#11437=DIRECTION('ref_axis',(-1.,0.,0.));
#11438=DIRECTION('',(0.,-1.,-1.04083408558608E-15));
#11439=DIRECTION('center_axis',(-1.,0.,0.));
#11440=DIRECTION('ref_axis',(0.,-1.,-1.04083408558608E-15));
#13523=CARTESIAN_POINT('',(0.,0.,0.));
#13524=CARTESIAN_POINT('Origin',(0.,0.0159712256101277,-0.012175853286558));
#13525=CARTESIAN_POINT('',(0.0028500000000131,0.0163712256101177,-0.012175853286558));
#13526=CARTESIAN_POINT('Origin',(0.,0.0163712256101177,-0.012175853286558));
#13527=CARTESIAN_POINT('',(0.00245000000001309,0.0159712256101177,-0.012175853286558));
#13528=CARTESIAN_POINT('Origin',(0.00285,0.0159712256101277,-0.012175853286558));
#13529=CARTESIAN_POINT('Origin',(0.,0.0159712256101177,-0.012175853286558));
#13530=CARTESIAN_POINT('Origin',(0.,0.0163712256101277,-0.012175853286558));
#13531=CARTESIAN_POINT('',(-0.00345,0.0163712256101177,-0.012175853286558));
#13532=CARTESIAN_POINT('Origin',(0.,0.0163712256101177,-0.012175853286558));
#13533=CARTESIAN_POINT('Origin',(0.,0.0163712256101277,-0.012175853286558));
#13534=CARTESIAN_POINT('',(0.00213600093632938,0.0129712256101277,-0.013375853286558));
#13535=CARTESIAN_POINT('',(0.00245,0.0129712256101177,-0.012175853286558));
#13536=CARTESIAN_POINT('Origin',(0.,0.0129712256101177,-0.012175853286558));
#13537=CARTESIAN_POINT('',(0.00213600093632938,0.0153712256101277,-0.013375853286558));
#13538=CARTESIAN_POINT('',(0.00213600093633938,0.0163712256101177,-0.013375853286568));
#13539=CARTESIAN_POINT('',(0.00095,0.0153712256101277,-0.0144341712446852));
#13540=CARTESIAN_POINT('Origin',(0.,0.0153712256101177,-0.012175853286558));
#13541=CARTESIAN_POINT('',(0.00095,0.0129712256101277,-0.0144341712446852));
#13542=CARTESIAN_POINT('',(0.00095000000001,0.0163712256101177,-0.0144341712446952));
#13543=CARTESIAN_POINT('',(-0.00095,0.0129712256101277,-0.0144341712446852));
#13544=CARTESIAN_POINT('Origin',(0.,0.0129712256101177,-0.012175853286558));
#13545=CARTESIAN_POINT('',(-0.00095,0.0153712256101277,-0.0144341712446852));
#13546=CARTESIAN_POINT('',(-0.00095000000001,0.0163712256101177,-0.0144341712446952));
#13547=CARTESIAN_POINT('',(-0.00213600093632938,0.0153712256101277,-0.013375853286558));
#13548=CARTESIAN_POINT('Origin',(0.,0.0153712256101177,-0.012175853286558));
#13549=CARTESIAN_POINT('',(-0.00213600093632938,0.0129712256101277,-0.013375853286558));
#13550=CARTESIAN_POINT('',(-0.00213600093633938,0.0163712256101177,-0.013375853286568));
#13551=CARTESIAN_POINT('',(-0.00213600093632938,0.0129712256101277,-0.010975853286558));
#13552=CARTESIAN_POINT('Origin',(0.,0.0129712256101177,-0.012175853286558));
#13553=CARTESIAN_POINT('',(-0.00213600093632938,0.0153712256101277,-0.010975853286558));
#13554=CARTESIAN_POINT('',(-0.00213600093633938,0.0163712256101177,-0.010975853286548));
#13555=CARTESIAN_POINT('',(-0.00095,0.0153712256101277,-0.00991753532843076));
#13556=CARTESIAN_POINT('Origin',(0.,0.0153712256101177,-0.012175853286558));
#13557=CARTESIAN_POINT('',(-0.00095,0.0129712256101277,-0.00991753532843077));
#13558=CARTESIAN_POINT('',(-0.00095000000001,0.0163712256101177,-0.00991753532842076));
#13559=CARTESIAN_POINT('',(0.00095,0.0129712256101277,-0.00991753532843077));
#13560=CARTESIAN_POINT('Origin',(0.,0.0129712256101177,-0.012175853286558));
#13561=CARTESIAN_POINT('',(0.00095,0.0153712256101277,-0.00991753532843076));
#13562=CARTESIAN_POINT('',(0.00095000000001,0.0163712256101177,-0.00991753532842076));
#13563=CARTESIAN_POINT('',(0.00213600093632938,0.0153712256101277,-0.010975853286558));
#13564=CARTESIAN_POINT('Origin',(0.,0.0153712256101177,-0.012175853286558));
#13565=CARTESIAN_POINT('',(0.00213600093632938,0.0129712256101277,-0.010975853286558));
#13566=CARTESIAN_POINT('',(0.00213600093633938,0.0163712256101177,-0.010975853286548));
#13567=CARTESIAN_POINT('Origin',(0.,0.0129712256101177,-0.012175853286558));
#13568=CARTESIAN_POINT('',(0.00245,0.0163712256101277,-0.012175853286558));
#13569=CARTESIAN_POINT('Origin',(0.,0.0171212256101277,-0.012175853286558));
#13570=CARTESIAN_POINT('',(0.00200000000001,0.0171212256101177,-0.012175853286558));
#13571=CARTESIAN_POINT('Origin',(0.,0.0171212256101177,-0.012175853286558));
#13572=CARTESIAN_POINT('',(0.00240000000001,0.0175212256101277,-0.012175853286558));
#13573=CARTESIAN_POINT('Origin',(0.0024,0.0171212256101277,-0.012175853286558));
#13574=CARTESIAN_POINT('Origin',(0.,0.0175212256101277,-0.012175853286558));
#13575=CARTESIAN_POINT('Origin',(0.,0.0129712256101277,-0.012175853286558));
#13576=CARTESIAN_POINT('',(0.002,0.0109712256101177,-0.012175853286558));
#13577=CARTESIAN_POINT('',(0.002,0.0129712256101277,-0.012175853286558));
#13578=CARTESIAN_POINT('',(0.0016,0.0109712256101277,-0.010975853286558));
#13579=CARTESIAN_POINT('Origin',(0.,0.0109712256101177,-0.012175853286558));
#13580=CARTESIAN_POINT('',(0.00151986841535707,0.0121712256101277,-0.010875853286558));
#13581=CARTESIAN_POINT('Origin',(0.,-0.0034287743898823,-0.012175853286558));
#13582=CARTESIAN_POINT('',(0.00151986841535707,0.0124712256101277,-0.010875853286558));
#13583=CARTESIAN_POINT('',(0.00151986841536707,0.0129712256101177,-0.010875853286548));
#13584=CARTESIAN_POINT('',(0.0016,0.0129712256101277,-0.010975853286558));
#13585=CARTESIAN_POINT('Origin',(0.,0.0189712256101377,-0.012175853286558));
#13586=CARTESIAN_POINT('',(0.0016,0.0153712256101277,-0.010975853286558));
#13587=CARTESIAN_POINT('',(0.00160000000001,0.0163712256101177,-0.010975853286548));
#13588=CARTESIAN_POINT('',(0.00095,0.0153712256101277,-0.0104158816958782));
#13589=CARTESIAN_POINT('Origin',(0.,0.0153712256101177,-0.012175853286558));
#13590=CARTESIAN_POINT('',(0.00095,0.0129712256101277,-0.0104158816958782));
#13591=CARTESIAN_POINT('',(0.00095000000001,0.0163712256101177,-0.0104158816958682));
#13592=CARTESIAN_POINT('',(0.00105,0.0124712256101277,-0.0104736488335031));
#13593=CARTESIAN_POINT('Origin',(0.,0.0177212256101377,-0.012175853286558));
#13594=CARTESIAN_POINT('',(0.00105,0.0121712256101277,-0.0104736488335031));
#13595=CARTESIAN_POINT('',(0.00105000000001,0.0129712256101177,-0.0104736488334931));
#13596=CARTESIAN_POINT('',(0.00095,0.0109712256101277,-0.0104158816958782));
#13597=CARTESIAN_POINT('Origin',(0.,-0.0004287743898823,-0.012175853286558));
#13598=CARTESIAN_POINT('',(-0.00095,0.0109712256101277,-0.0104158816958782));
#13599=CARTESIAN_POINT('Origin',(0.,0.0109712256101177,-0.012175853286558));
#13600=CARTESIAN_POINT('',(-0.00105,0.0121712256101277,-0.0104736488335031));
#13601=CARTESIAN_POINT('Origin',(0.,-0.0004287743898823,-0.012175853286558));
#13602=CARTESIAN_POINT('',(-0.00105,0.0124712256101277,-0.0104736488335031));
#13603=CARTESIAN_POINT('',(-0.00105000000001,0.0129712256101177,-0.0104736488334931));
#13604=CARTESIAN_POINT('',(-0.00095,0.0129712256101277,-0.0104158816958782));
#13605=CARTESIAN_POINT('Origin',(0.,0.0177212256101377,-0.012175853286558));
#13606=CARTESIAN_POINT('',(-0.00095,0.0153712256101277,-0.0104158816958782));
#13607=CARTESIAN_POINT('',(-0.00095000000001,0.0163712256101177,-0.0104158816958682));
#13608=CARTESIAN_POINT('',(-0.0016,0.0153712256101277,-0.010975853286558));
#13609=CARTESIAN_POINT('Origin',(0.,0.0153712256101177,-0.012175853286558));
#13610=CARTESIAN_POINT('',(-0.0016,0.0129712256101277,-0.010975853286558));
#13611=CARTESIAN_POINT('',(-0.00160000000001,0.0163712256101177,-0.010975853286548));
#13612=CARTESIAN_POINT('',(-0.00151986841535707,0.0124712256101277,-0.010875853286558));
#13613=CARTESIAN_POINT('Origin',(0.,0.0189712256101377,-0.012175853286558));
#13614=CARTESIAN_POINT('',(-0.00151986841535707,0.0121712256101277,-0.010875853286558));
#13615=CARTESIAN_POINT('',(-0.00151986841536707,0.0129712256101177,-0.010875853286548));
#13616=CARTESIAN_POINT('',(-0.0016,0.0109712256101277,-0.010975853286558));
#13617=CARTESIAN_POINT('Origin',(0.,-0.0034287743898823,-0.012175853286558));
#13618=CARTESIAN_POINT('',(-0.0016,0.0109712256101277,-0.013375853286558));
#13619=CARTESIAN_POINT('Origin',(0.,0.0109712256101177,-0.012175853286558));
#13620=CARTESIAN_POINT('',(-0.00151986841535707,0.0121712256101277,-0.013475853286558));
#13621=CARTESIAN_POINT('Origin',(0.,-0.0034287743898823,-0.012175853286558));
#13622=CARTESIAN_POINT('',(-0.00151986841535707,0.0124712256101277,-0.013475853286558));
#13623=CARTESIAN_POINT('',(-0.00151986841536707,0.0129712256101177,-0.013475853286568));
#13624=CARTESIAN_POINT('',(-0.0016,0.0129712256101277,-0.013375853286558));
#13625=CARTESIAN_POINT('Origin',(0.,0.0189712256101377,-0.012175853286558));
#13626=CARTESIAN_POINT('',(-0.0016,0.0153712256101277,-0.013375853286558));
#13627=CARTESIAN_POINT('',(-0.00160000000001,0.0163712256101177,-0.013375853286568));
#13628=CARTESIAN_POINT('',(-0.00095,0.0153712256101277,-0.0139358248772378));
#13629=CARTESIAN_POINT('Origin',(0.,0.0153712256101177,-0.012175853286558));
#13630=CARTESIAN_POINT('',(-0.00095,0.0129712256101277,-0.0139358248772378));
#13631=CARTESIAN_POINT('',(-0.00095000000001,0.0163712256101177,-0.0139358248772478));
#13632=CARTESIAN_POINT('',(-0.00105,0.0124712256101277,-0.0138780577396129));
#13633=CARTESIAN_POINT('Origin',(0.,0.0177212256101377,-0.012175853286558));
#13634=CARTESIAN_POINT('',(-0.00105,0.0121712256101277,-0.0138780577396129));
#13635=CARTESIAN_POINT('',(-0.00105000000001,0.0129712256101177,-0.0138780577396229));
#13636=CARTESIAN_POINT('',(-0.00095,0.0109712256101277,-0.0139358248772378));
#13637=CARTESIAN_POINT('Origin',(0.,-0.0004287743898823,-0.012175853286558));
#13638=CARTESIAN_POINT('',(0.00095,0.0109712256101277,-0.0139358248772378));
#13639=CARTESIAN_POINT('Origin',(0.,0.0109712256101177,-0.012175853286558));
#13640=CARTESIAN_POINT('',(0.00105,0.0121712256101277,-0.0138780577396129));
#13641=CARTESIAN_POINT('Origin',(0.,-0.0004287743898823,-0.012175853286558));
#13642=CARTESIAN_POINT('',(0.00105,0.0124712256101277,-0.0138780577396129));
#13643=CARTESIAN_POINT('',(0.00105000000001,0.0129712256101177,-0.0138780577396229));
#13644=CARTESIAN_POINT('',(0.00095,0.0129712256101277,-0.0139358248772378));
#13645=CARTESIAN_POINT('Origin',(0.,0.0177212256101377,-0.012175853286558));
#13646=CARTESIAN_POINT('',(0.00095,0.0153712256101277,-0.0139358248772378));
#13647=CARTESIAN_POINT('',(0.00095000000001,0.0163712256101177,-0.0139358248772478));
#13648=CARTESIAN_POINT('',(0.0016,0.0153712256101277,-0.013375853286558));
#13649=CARTESIAN_POINT('Origin',(0.,0.0153712256101177,-0.012175853286558));
#13650=CARTESIAN_POINT('',(0.0016,0.0129712256101277,-0.013375853286558));
#13651=CARTESIAN_POINT('',(0.00160000000001,0.0163712256101177,-0.013375853286568));
#13652=CARTESIAN_POINT('',(0.00151986841535707,0.0124712256101277,-0.013475853286558));
#13653=CARTESIAN_POINT('Origin',(0.,0.0189712256101377,-0.012175853286558));
#13654=CARTESIAN_POINT('',(0.00151986841535707,0.0121712256101277,-0.013475853286558));
#13655=CARTESIAN_POINT('',(0.00151986841536707,0.0129712256101177,-0.013475853286568));
#13656=CARTESIAN_POINT('',(0.0016,0.0109712256101277,-0.013375853286558));
#13657=CARTESIAN_POINT('Origin',(0.,-0.0034287743898823,-0.012175853286558));
#13658=CARTESIAN_POINT('Origin',(0.,0.0109712256101177,-0.012175853286558));
#13659=CARTESIAN_POINT('Origin',(0.,0.0175212256101277,-0.012175853286558));
#13660=CARTESIAN_POINT('',(-0.00345,0.0175212256101277,-0.012175853286558));
#13661=CARTESIAN_POINT('Origin',(0.,0.0175212256101277,-0.012175853286558));
#13662=CARTESIAN_POINT('Origin',(0.001,0.0115712256101277,-0.0143575051632916));
#13663=CARTESIAN_POINT('',(0.00095,0.0109712256101277,-0.0143252718125785));
#13664=CARTESIAN_POINT('',(0.00095000000001,0.0109712256101177,-0.0143575051633016));
#13665=CARTESIAN_POINT('',(0.00105,0.0121712256101277,-0.0148253815464564));
#13666=CARTESIAN_POINT('Ctrl Pts',(0.00095000000001,0.0109712256101177,
-0.0143252718125885));
#13667=CARTESIAN_POINT('Ctrl Pts',(0.000994789380303646,0.0115086981736415,
-0.014550321192835));
#13668=CARTESIAN_POINT('Ctrl Pts',(0.00105000000001,0.0121712256101177,
-0.0148253815464664));
#13669=CARTESIAN_POINT('',(0.00105000000001,0.0121712256101177,-0.0143575051633016));
#13670=CARTESIAN_POINT('Origin',(0.,0.0115712256101277,-0.012175853286558));
#13671=CARTESIAN_POINT('',(-0.00095,0.0109712256101277,-0.0143252718125785));
#13672=CARTESIAN_POINT('Origin',(0.,0.0109712256101177,-0.012175853286558));
#13673=CARTESIAN_POINT('',(-0.00105,0.0121712256101277,-0.0148253815464564));
#13674=CARTESIAN_POINT('Ctrl Pts',(-0.00105000000001,0.0121712256101177,
-0.0148253815464664));
#13675=CARTESIAN_POINT('Ctrl Pts',(-0.000994789380303646,0.0115086981736415,
-0.014550321192835));
#13676=CARTESIAN_POINT('Ctrl Pts',(-0.00095000000001,0.0109712256101177,
-0.0143252718125885));
#13677=CARTESIAN_POINT('Origin',(0.,0.0121712256101177,-0.012175853286558));
#13678=CARTESIAN_POINT('Origin',(1.38777878078145E-19,0.0109712256101277,
-0.0142808390818979));
#13679=CARTESIAN_POINT('',(-0.00095000000001,0.0109712256101177,-0.0141083319795779));
#13680=CARTESIAN_POINT('Origin',(-0.001,0.0115712256101277,-0.0141083319795679));
#13681=CARTESIAN_POINT('',(-0.00105000000001,0.0121712256101177,-0.0141083319795779));
#13682=CARTESIAN_POINT('Origin',(-0.00208050046816469,0.0115712256101277,
-0.013425853286558));
#13683=CARTESIAN_POINT('',(-0.00202051973511768,0.0109712256101277,-0.013375853286558));
#13684=CARTESIAN_POINT('',(-0.00208050046817469,0.0109712256101177,-0.013375853286568));
#13685=CARTESIAN_POINT('',(-0.00253623737059448,0.0121712256101277,-0.013475853286558));
#13686=CARTESIAN_POINT('Ctrl Pts',(-0.00202051973512767,0.0109712256101177,
-0.013375853286568));
#13687=CARTESIAN_POINT('Ctrl Pts',(-0.00225204403530932,0.0115033197344889,
-0.0134201944635989));
#13688=CARTESIAN_POINT('Ctrl Pts',(-0.00253623737060448,0.0121712256101177,
-0.013475853286568));
#13689=CARTESIAN_POINT('',(-0.00208050046817469,0.0121712256101177,-0.013475853286568));
#13690=CARTESIAN_POINT('Origin',(-0.002025,0.0109712256101277,-0.012175853286558));
#13691=CARTESIAN_POINT('',(-0.00202051973511768,0.0109712256101277,-0.010975853286558));
#13692=CARTESIAN_POINT('',(-0.00181250000001,0.0109712256101177,-0.010975853286548));
#13693=CARTESIAN_POINT('Origin',(0.,0.0109712256101177,-0.012175853286558));
#13694=CARTESIAN_POINT('Origin',(0.0018125,0.0115712256101277,-0.013425853286558));
#13695=CARTESIAN_POINT('',(0.00253623737059448,0.0121712256101277,-0.013475853286558));
#13696=CARTESIAN_POINT('',(0.00202051973511768,0.0109712256101277,-0.013375853286558));
#13697=CARTESIAN_POINT('Ctrl Pts',(0.00253623737060448,0.0121712256101177,
-0.013475853286568));
#13698=CARTESIAN_POINT('Ctrl Pts',(0.00225204403530932,0.0115033197344889,
-0.0134201944635989));
#13699=CARTESIAN_POINT('Ctrl Pts',(0.00202051973512767,0.0109712256101177,
-0.013375853286568));
#13700=CARTESIAN_POINT('',(0.00181250000001,0.0109712256101177,-0.013375853286568));
#13701=CARTESIAN_POINT('',(0.00181250000001,0.0121712256101177,-0.013475853286568));
#13702=CARTESIAN_POINT('Origin',(0.002025,0.0109712256101277,-0.012175853286558));
#13703=CARTESIAN_POINT('',(0.00202051973511768,0.0109712256101277,-0.010975853286558));
#13704=CARTESIAN_POINT('Origin',(0.,0.0109712256101177,-0.012175853286558));
#13705=CARTESIAN_POINT('',(0.00208050046817469,0.0109712256101177,-0.010975853286548));
#13706=CARTESIAN_POINT('Origin',(0.00208050046816469,0.0115712256101277,
-0.010925853286558));
#13707=CARTESIAN_POINT('',(0.00253623737059448,0.0121712256101277,-0.010875853286558));
#13708=CARTESIAN_POINT('Ctrl Pts',(0.00202051973512767,0.0109712256101177,
-0.010975853286548));
#13709=CARTESIAN_POINT('Ctrl Pts',(0.00225204403530932,0.0115033197344889,
-0.0109315121095171));
#13710=CARTESIAN_POINT('Ctrl Pts',(0.00253623737060448,0.0121712256101177,
-0.010875853286548));
#13711=CARTESIAN_POINT('',(0.00208050046817469,0.0121712256101177,-0.010875853286548));
#13712=CARTESIAN_POINT('Origin',(0.001,0.0115712256101277,-0.0102433745935482));
#13713=CARTESIAN_POINT('',(0.00105,0.0121712256101277,-0.00952632502665966));
#13714=CARTESIAN_POINT('',(0.00095,0.0109712256101277,-0.0100264347605375));
#13715=CARTESIAN_POINT('Ctrl Pts',(0.00105000000001,0.0121712256101177,
-0.00952632502664966));
#13716=CARTESIAN_POINT('Ctrl Pts',(0.000994789380303646,0.0115086981736415,
-0.00980138538028098));
#13717=CARTESIAN_POINT('Ctrl Pts',(0.00095000000001,0.0109712256101177,
-0.0100264347605275));
#13718=CARTESIAN_POINT('',(0.00095000000001,0.0109712256101177,-0.0102433745935382));
#13719=CARTESIAN_POINT('',(0.00105000000001,0.0121712256101177,-0.0102433745935382));
#13720=CARTESIAN_POINT('Origin',(1.38777878078145E-19,0.0109712256101277,
-0.0100708674912181));
#13721=CARTESIAN_POINT('',(-0.00095,0.0109712256101277,-0.0100264347605375));
#13722=CARTESIAN_POINT('Origin',(0.,0.0109712256101177,-0.012175853286558));
#13723=CARTESIAN_POINT('',(-0.00095000000001,0.0109712256101177,-0.00999420140981444));
#13724=CARTESIAN_POINT('Origin',(0.,0.0115712256101277,-0.012175853286558));
#13725=CARTESIAN_POINT('',(-0.00105,0.0121712256101277,-0.00952632502665966));
#13726=CARTESIAN_POINT('Origin',(0.,0.0121712256101177,-0.012175853286558));
#13727=CARTESIAN_POINT('Ctrl Pts',(-0.00095000000001,0.0109712256101177,
-0.0100264347605275));
#13728=CARTESIAN_POINT('Ctrl Pts',(-0.000994789380303646,0.0115086981736415,
-0.00980138538028098));
#13729=CARTESIAN_POINT('Ctrl Pts',(-0.00105000000001,0.0121712256101177,
-0.00952632502664966));
#13730=CARTESIAN_POINT('Origin',(-0.0018125,0.0115712256101277,-0.010925853286558));
#13731=CARTESIAN_POINT('',(-0.00253623737059448,0.0121712256101277,-0.010875853286558));
#13732=CARTESIAN_POINT('Ctrl Pts',(-0.00253623737060448,0.0121712256101177,
-0.010875853286548));
#13733=CARTESIAN_POINT('Ctrl Pts',(-0.00225204403530932,0.0115033197344889,
-0.0109315121095171));
#13734=CARTESIAN_POINT('Ctrl Pts',(-0.00202051973512767,0.0109712256101177,
-0.010975853286548));
#13735=CARTESIAN_POINT('',(-0.00181250000001,0.0121712256101177,-0.010875853286548));
#13736=CARTESIAN_POINT('Origin',(0.,0.0115712256101277,-0.012175853286558));
#13737=CARTESIAN_POINT('Origin',(0.,0.0121712256101177,-0.012175853286558));
#13738=CARTESIAN_POINT('Origin',(-0.001,0.0115712256101277,-0.00999420140982444));
#13739=CARTESIAN_POINT('',(-0.00105000000001,0.0121712256101177,-0.00999420140981444));
#13740=CARTESIAN_POINT('Origin',(-0.00105,0.0129712256101277,-0.00991753532843077));
#13741=CARTESIAN_POINT('',(-0.00105,0.0124712256101277,-0.00952632502665966));
#13742=CARTESIAN_POINT('',(-0.00105000000001,0.0129712256101177,-0.00952632502664966));
#13743=CARTESIAN_POINT('',(-0.00105000000001,0.0124712256101177,-0.00999420140981444));
#13744=CARTESIAN_POINT('Origin',(-0.00208050046816469,0.0127212256101277,
-0.013425853286558));
#13745=CARTESIAN_POINT('',(-0.00253623737059448,0.0124712256101277,-0.013475853286558));
#13746=CARTESIAN_POINT('',(-0.00208050046817469,0.0124712256101177,-0.013475853286568));
#13747=CARTESIAN_POINT('',(-0.00225,0.0129712256101277,-0.013375853286558));
#13748=CARTESIAN_POINT('Origin',(0.417653699675352,-0.218496268260033,-0.0596693520771347));
#13749=CARTESIAN_POINT('',(-0.00208050046817469,0.0129712256101177,-0.013375853286568));
#13750=CARTESIAN_POINT('',(-0.00208050046817469,0.0129712256101177,-0.013375853286568));
#13751=CARTESIAN_POINT('Origin',(-0.002025,0.0129712256101277,-0.012175853286558));
#13752=CARTESIAN_POINT('',(-0.00225,0.0129712256101277,-0.010975853286558));
#13753=CARTESIAN_POINT('Origin',(0.,0.0129712256101177,-0.012175853286558));
#13754=CARTESIAN_POINT('',(-0.00181250000001,0.0129712256101177,-0.010975853286548));
#13755=CARTESIAN_POINT('Origin',(0.,0.0127212256101277,-0.012175853286558));
#13756=CARTESIAN_POINT('',(-0.00253623737059448,0.0124712256101277,-0.010875853286558));
#13757=CARTESIAN_POINT('Origin',(0.,0.0124712256101177,-0.012175853286558));
#13758=CARTESIAN_POINT('Origin',(0.417653699675352,-0.218496268260033,0.0353176455040183));
#13759=CARTESIAN_POINT('Origin',(-0.001,0.0127212256101277,-0.0141083319795679));
#13760=CARTESIAN_POINT('',(-0.00095,0.0129712256101277,-0.0145422851997979));
#13761=CARTESIAN_POINT('',(-0.00105,0.0124712256101277,-0.0148253815464564));
#13762=CARTESIAN_POINT('Ctrl Pts',(-0.000950000000000006,0.0129712256101277,
-0.0145422851997978));
#13763=CARTESIAN_POINT('Ctrl Pts',(-0.000997178044325374,0.0127353353885008,
-0.0146758588281839));
#13764=CARTESIAN_POINT('Ctrl Pts',(-0.00105,0.0124712256101277,-0.0148253815464564));
#13765=CARTESIAN_POINT('',(-0.00105000000001,0.0124712256101177,-0.0141083319795779));
#13766=CARTESIAN_POINT('',(-0.00095000000001,0.0129712256101177,-0.0141083319795779));
#13767=CARTESIAN_POINT('',(-0.00095000000001,0.0129712256101177,-0.0141083319795779));
#13768=CARTESIAN_POINT('Origin',(0.,0.0127212256101277,-0.012175853286558));
#13769=CARTESIAN_POINT('',(0.00095,0.0129712256101277,-0.0145422851997979));
#13770=CARTESIAN_POINT('Origin',(0.,0.0129712256101177,-0.012175853286558));
#13771=CARTESIAN_POINT('',(0.00105,0.0124712256101277,-0.0148253815464564));
#13772=CARTESIAN_POINT('Ctrl Pts',(0.00105,0.0124712256101277,-0.0148253815464564));
#13773=CARTESIAN_POINT('Ctrl Pts',(0.000997178044325414,0.0127353353885006,
-0.0146758588281841));
#13774=CARTESIAN_POINT('Ctrl Pts',(0.000950000000000005,0.0129712256101277,
-0.0145422851997979));
#13775=CARTESIAN_POINT('Origin',(0.,0.0124712256101177,-0.012175853286558));
#13776=CARTESIAN_POINT('Origin',(1.38777878078145E-19,0.0129712256101277,
-0.0142808390818979));
#13777=CARTESIAN_POINT('',(0.00095000000001,0.0129712256101177,-0.0143575051633016));
#13778=CARTESIAN_POINT('Origin',(0.001,0.0127212256101277,-0.0143575051632916));
#13779=CARTESIAN_POINT('',(0.00105000000001,0.0124712256101177,-0.0143575051633016));
#13780=CARTESIAN_POINT('',(0.00095000000001,0.0129712256101177,-0.0143575051633016));
#13781=CARTESIAN_POINT('Origin',(0.00105,0.0129712256101277,-0.0144341712446852));
#13782=CARTESIAN_POINT('',(0.00105000000001,0.0129712256101177,-0.0148253815464664));
#13783=CARTESIAN_POINT('Origin',(0.0018125,0.0127212256101277,-0.013425853286558));
#13784=CARTESIAN_POINT('',(0.00225,0.0129712256101277,-0.013375853286558));
#13785=CARTESIAN_POINT('',(0.00253623737059448,0.0124712256101277,-0.013475853286558));
#13786=CARTESIAN_POINT('Origin',(-0.417653699675352,-0.218496268260033,
-0.0596693520771347));
#13787=CARTESIAN_POINT('',(0.00181250000001,0.0124712256101177,-0.013475853286568));
#13788=CARTESIAN_POINT('',(0.00181250000001,0.0129712256101177,-0.013375853286568));
#13789=CARTESIAN_POINT('',(0.00181250000001,0.0129712256101177,-0.013375853286568));
#13790=CARTESIAN_POINT('Origin',(0.,0.0127212256101277,-0.012175853286558));
#13791=CARTESIAN_POINT('',(0.00225,0.0129712256101277,-0.010975853286558));
#13792=CARTESIAN_POINT('Origin',(0.,0.0129712256101177,-0.012175853286558));
#13793=CARTESIAN_POINT('',(0.00253623737059448,0.0124712256101277,-0.010875853286558));
#13794=CARTESIAN_POINT('Origin',(-0.417653699675352,-0.218496268260033,
0.0353176455040183));
#13795=CARTESIAN_POINT('Origin',(0.,0.0124712256101177,-0.012175853286558));
#13796=CARTESIAN_POINT('Origin',(0.002025,0.0129712256101277,-0.012175853286558));
#13797=CARTESIAN_POINT('',(0.00208050046817469,0.0129712256101177,-0.010975853286548));
#13798=CARTESIAN_POINT('Origin',(0.00208050046816469,0.0127212256101277,
-0.010925853286558));
#13799=CARTESIAN_POINT('',(0.00208050046817469,0.0124712256101177,-0.010875853286548));
#13800=CARTESIAN_POINT('',(0.00208050046817469,0.0129712256101177,-0.010975853286548));
#13801=CARTESIAN_POINT('Origin',(0.00213600093632938,0.0129712256101277,
-0.010875853286558));
#13802=CARTESIAN_POINT('',(0.00253623737060448,0.0129712256101177,-0.010875853286548));
#13803=CARTESIAN_POINT('Origin',(0.001,0.0127212256101277,-0.0102433745935482));
#13804=CARTESIAN_POINT('',(0.00095,0.0129712256101277,-0.00980942137331815));
#13805=CARTESIAN_POINT('',(0.00105,0.0124712256101277,-0.00952632502665966));
#13806=CARTESIAN_POINT('Ctrl Pts',(0.00095,0.0129712256101277,-0.00980942137331815));
#13807=CARTESIAN_POINT('Ctrl Pts',(0.000997178044311125,0.0127353353885721,
-0.00967584774497245));
#13808=CARTESIAN_POINT('Ctrl Pts',(0.00105,0.0124712256101277,-0.00952632502665967));
#13809=CARTESIAN_POINT('',(0.00105000000001,0.0124712256101177,-0.0102433745935382));
#13810=CARTESIAN_POINT('',(0.00095000000001,0.0129712256101177,-0.0102433745935382));
#13811=CARTESIAN_POINT('',(0.00095000000001,0.0129712256101177,-0.0102433745935382));
#13812=CARTESIAN_POINT('Origin',(0.,0.0127212256101277,-0.012175853286558));
#13813=CARTESIAN_POINT('',(-0.00095,0.0129712256101277,-0.00980942137331815));
#13814=CARTESIAN_POINT('Origin',(0.,0.0129712256101177,-0.012175853286558));
#13815=CARTESIAN_POINT('Ctrl Pts',(-0.00104999999999999,0.0124712256101277,
-0.00952632502665963));
#13816=CARTESIAN_POINT('Ctrl Pts',(-0.000997178044319801,0.0127353353885287,
-0.00967584774494786));
#13817=CARTESIAN_POINT('Ctrl Pts',(-0.00095,0.0129712256101277,-0.00980942137331816));
#13818=CARTESIAN_POINT('Origin',(0.,0.0124712256101177,-0.012175853286558));
#13819=CARTESIAN_POINT('Origin',(1.38777878078145E-19,0.0129712256101277,
-0.0100708674912181));
#13820=CARTESIAN_POINT('',(-0.00095000000001,0.0129712256101177,-0.00999420140981443));
#13821=CARTESIAN_POINT('Origin',(-0.0018125,0.0127212256101277,-0.010925853286558));
#13822=CARTESIAN_POINT('',(-0.00181250000001,0.0124712256101177,-0.010875853286548));
#13823=CARTESIAN_POINT('',(-0.00181250000001,0.0129712256101177,-0.010975853286548));
#13824=CARTESIAN_POINT('Origin',(-0.001,0.0127212256101277,-0.00999420140982444));
#13825=CARTESIAN_POINT('',(-0.00095000000001,0.0129712256101177,-0.00999420140981443));
#13826=CARTESIAN_POINT('Origin',(-0.00095,0.0163712256101277,-0.0139358248772378));
#13827=CARTESIAN_POINT('',(-0.00095000000001,0.0153712256101177,-0.0144341712446952));
#13828=CARTESIAN_POINT('Origin',(0.00095,0.0163712256101277,-0.0144341712446852));
#13829=CARTESIAN_POINT('',(0.00095000000001,0.0153712256101177,-0.0139358248772478));
#13830=CARTESIAN_POINT('Origin',(-0.0016,0.0163712256101277,-0.010975853286558));
#13831=CARTESIAN_POINT('',(-0.00213600093633938,0.0153712256101177,-0.010975853286548));
#13832=CARTESIAN_POINT('Origin',(-0.00213600093632938,0.0163712256101277,
-0.013375853286558));
#13833=CARTESIAN_POINT('',(-0.00160000000001,0.0153712256101177,-0.013375853286568));
#13834=CARTESIAN_POINT('Origin',(0.0016,0.0163712256101277,-0.013375853286558));
#13835=CARTESIAN_POINT('',(0.00213600093633938,0.0153712256101177,-0.013375853286568));
#13836=CARTESIAN_POINT('Origin',(0.00213600093632938,0.0163712256101277,
-0.010975853286558));
#13837=CARTESIAN_POINT('',(0.00160000000001,0.0153712256101177,-0.010975853286548));
#13838=CARTESIAN_POINT('Origin',(0.00095,0.0163712256101277,-0.0104158816958782));
#13839=CARTESIAN_POINT('',(0.00095000000001,0.0153712256101177,-0.00991753532842076));
#13840=CARTESIAN_POINT('Origin',(-0.00095,0.0163712256101277,-0.00991753532843076));
#13841=CARTESIAN_POINT('',(-0.00095000000001,0.0153712256101177,-0.0104158816958682));
#13842=CARTESIAN_POINT('Origin',(-0.00154300046816469,0.0153712256101277,
-0.0139050122656216));
#13843=CARTESIAN_POINT('Origin',(-0.00154300046816469,0.0153712256101277,
-0.0104466943074944));
#13844=CARTESIAN_POINT('Origin',(0.00154300046816469,0.0153712256101277,
-0.0139050122656216));
#13845=CARTESIAN_POINT('Origin',(0.00154300046816469,0.0153712256101277,
-0.0104466943074944));
#13846=CARTESIAN_POINT('Origin',(0.,0.0175212256101277,-0.012175853286558));
#13847=CARTESIAN_POINT('',(-0.00345,0.0175212256101277,-0.012175853286558));
#13848=CARTESIAN_POINT('Origin',(-0.00213600093632938,0.0129712256101277,
-0.013475853286558));
#13849=CARTESIAN_POINT('',(-0.00253623737060448,0.0129712256101177,-0.013475853286568));
#13850=CARTESIAN_POINT('Origin',(0.,0.0129712256101277,-0.012175853286558));
#13851=CARTESIAN_POINT('',(-0.00253623737060448,0.0129712256101177,-0.010875853286548));
#13852=CARTESIAN_POINT('Origin',(-0.0016,0.0129712256101277,-0.010875853286558));
#13853=CARTESIAN_POINT('Origin',(0.,0.0115712256101277,-0.012175853286558));
#13854=CARTESIAN_POINT('Origin',(0.,0.0121712256101177,-0.012175853286558));
#13855=CARTESIAN_POINT('Origin',(0.,0.0129712256101277,-0.012175853286558));
#13856=CARTESIAN_POINT('',(0.00253623737060448,0.0129712256101177,-0.013475853286568));
#13857=CARTESIAN_POINT('Origin',(0.0016,0.0129712256101277,-0.013475853286558));
#13858=CARTESIAN_POINT('Origin',(0.,0.0129712256101277,-0.012175853286558));
#13859=CARTESIAN_POINT('',(0.00105000000001,0.0129712256101177,-0.00952632502664966));
#13860=CARTESIAN_POINT('Origin',(0.00105,0.0129712256101277,-0.0104158816958782));
#13861=CARTESIAN_POINT('Origin',(0.,0.0129712256101277,-0.012175853286558));
#13862=CARTESIAN_POINT('',(-0.00105000000001,0.0129712256101177,-0.0148253815464664));
#13863=CARTESIAN_POINT('Origin',(-0.00105,0.0129712256101277,-0.0139358248772378));
#50042=UNCERTAINTY_MEASURE_WITH_UNIT(LENGTH_MEASURE(1.E-5),#50082,
'DISTANCE_ACCURACY_VALUE',
'Maximum model space distance between geometric entities at asserted c
onnectivities');
#50059=UNCERTAINTY_MEASURE_WITH_UNIT(LENGTH_MEASURE(1.E-5),#50082,
'DISTANCE_ACCURACY_VALUE',
'Maximum model space distance between geometric entities at asserted c
onnectivities');
#50064=(
GEOMETRIC_REPRESENTATION_CONTEXT(3)
GLOBAL_UNCERTAINTY_ASSIGNED_CONTEXT((#50042))
GLOBAL_UNIT_ASSIGNED_CONTEXT((#50082,#50083,#50084))
REPRESENTATION_CONTEXT('','3D')
);
#50081=(
GEOMETRIC_REPRESENTATION_CONTEXT(3)
GLOBAL_UNCERTAINTY_ASSIGNED_CONTEXT((#50059))
GLOBAL_UNIT_ASSIGNED_CONTEXT((#50082,#50083,#50084))
REPRESENTATION_CONTEXT('','3D')
);
#50082=(
LENGTH_UNIT()
NAMED_UNIT(*)
SI_UNIT($,.METRE.)
);
#50083=(
NAMED_UNIT(*)
PLANE_ANGLE_UNIT()
SI_UNIT($,.RADIAN.)
);
#50084=(
NAMED_UNIT(*)
SI_UNIT($,.STERADIAN.)
SOLID_ANGLE_UNIT()
);
#50089=SHAPE_DEFINITION_REPRESENTATION(#50110,#50151);
#50110=PRODUCT_DEFINITION_SHAPE('',$,#50173);
#50151=SHAPE_REPRESENTATION('',(#10139),#50064);
#50168=PRODUCT_DEFINITION_CONTEXT('part definition',#50233,'design');
#50173=PRODUCT_DEFINITION('Tube coupler','Tube coupler',#50194,#50168);
#50194=PRODUCT_DEFINITION_FORMATION('',$,#50239);
#50233=APPLICATION_CONTEXT('Managed model based 3d engineering');
#50234=PRODUCT_CONTEXT('part definition',#50233,'mechanical');
#50239=PRODUCT('Tube coupler','Tube coupler',
'LEGAL AND USAGE DISCLAIMER: this Data/Model is provided \X2\201C\X0\A
S IS\X2\201D\X0\ for informational and representational only. It is a 
geometric approximation and is NOT engineered, certified, or guarantee
d for dimensional accuracy, exact tolerances, or production-level prec
ision. Vendor disclaims all implied warranties including fitness for a
 particular purpose. DO NOT USE FOR DIRECT PHYSICAL MANUFACTURING, AUT
OMATED PRODUCTION, OR SAFETY-CRITICAL SYSTEMS without independent engi
neering verification and resolution of any design discrepancies.',(#50234));
#50260=PRESENTATION_STYLE_ASSIGNMENT((#50267));
#50267=SURFACE_STYLE_USAGE(.BOTH.,#50274);
#50274=SURFACE_SIDE_STYLE('',(#50281));
#50281=SURFACE_STYLE_FILL_AREA(#50288);
#50288=FILL_AREA_STYLE('Opaque(25,25,25)',(#50295));
#50295=FILL_AREA_STYLE_COLOUR('Opaque(25,25,25)',#50302);
#50302=COLOUR_RGB('Opaque(25,25,25)',0.0980392156862745,0.0980392156862745,
0.0980392156862745);
ENDSEC;
END-ISO-10303-21;
